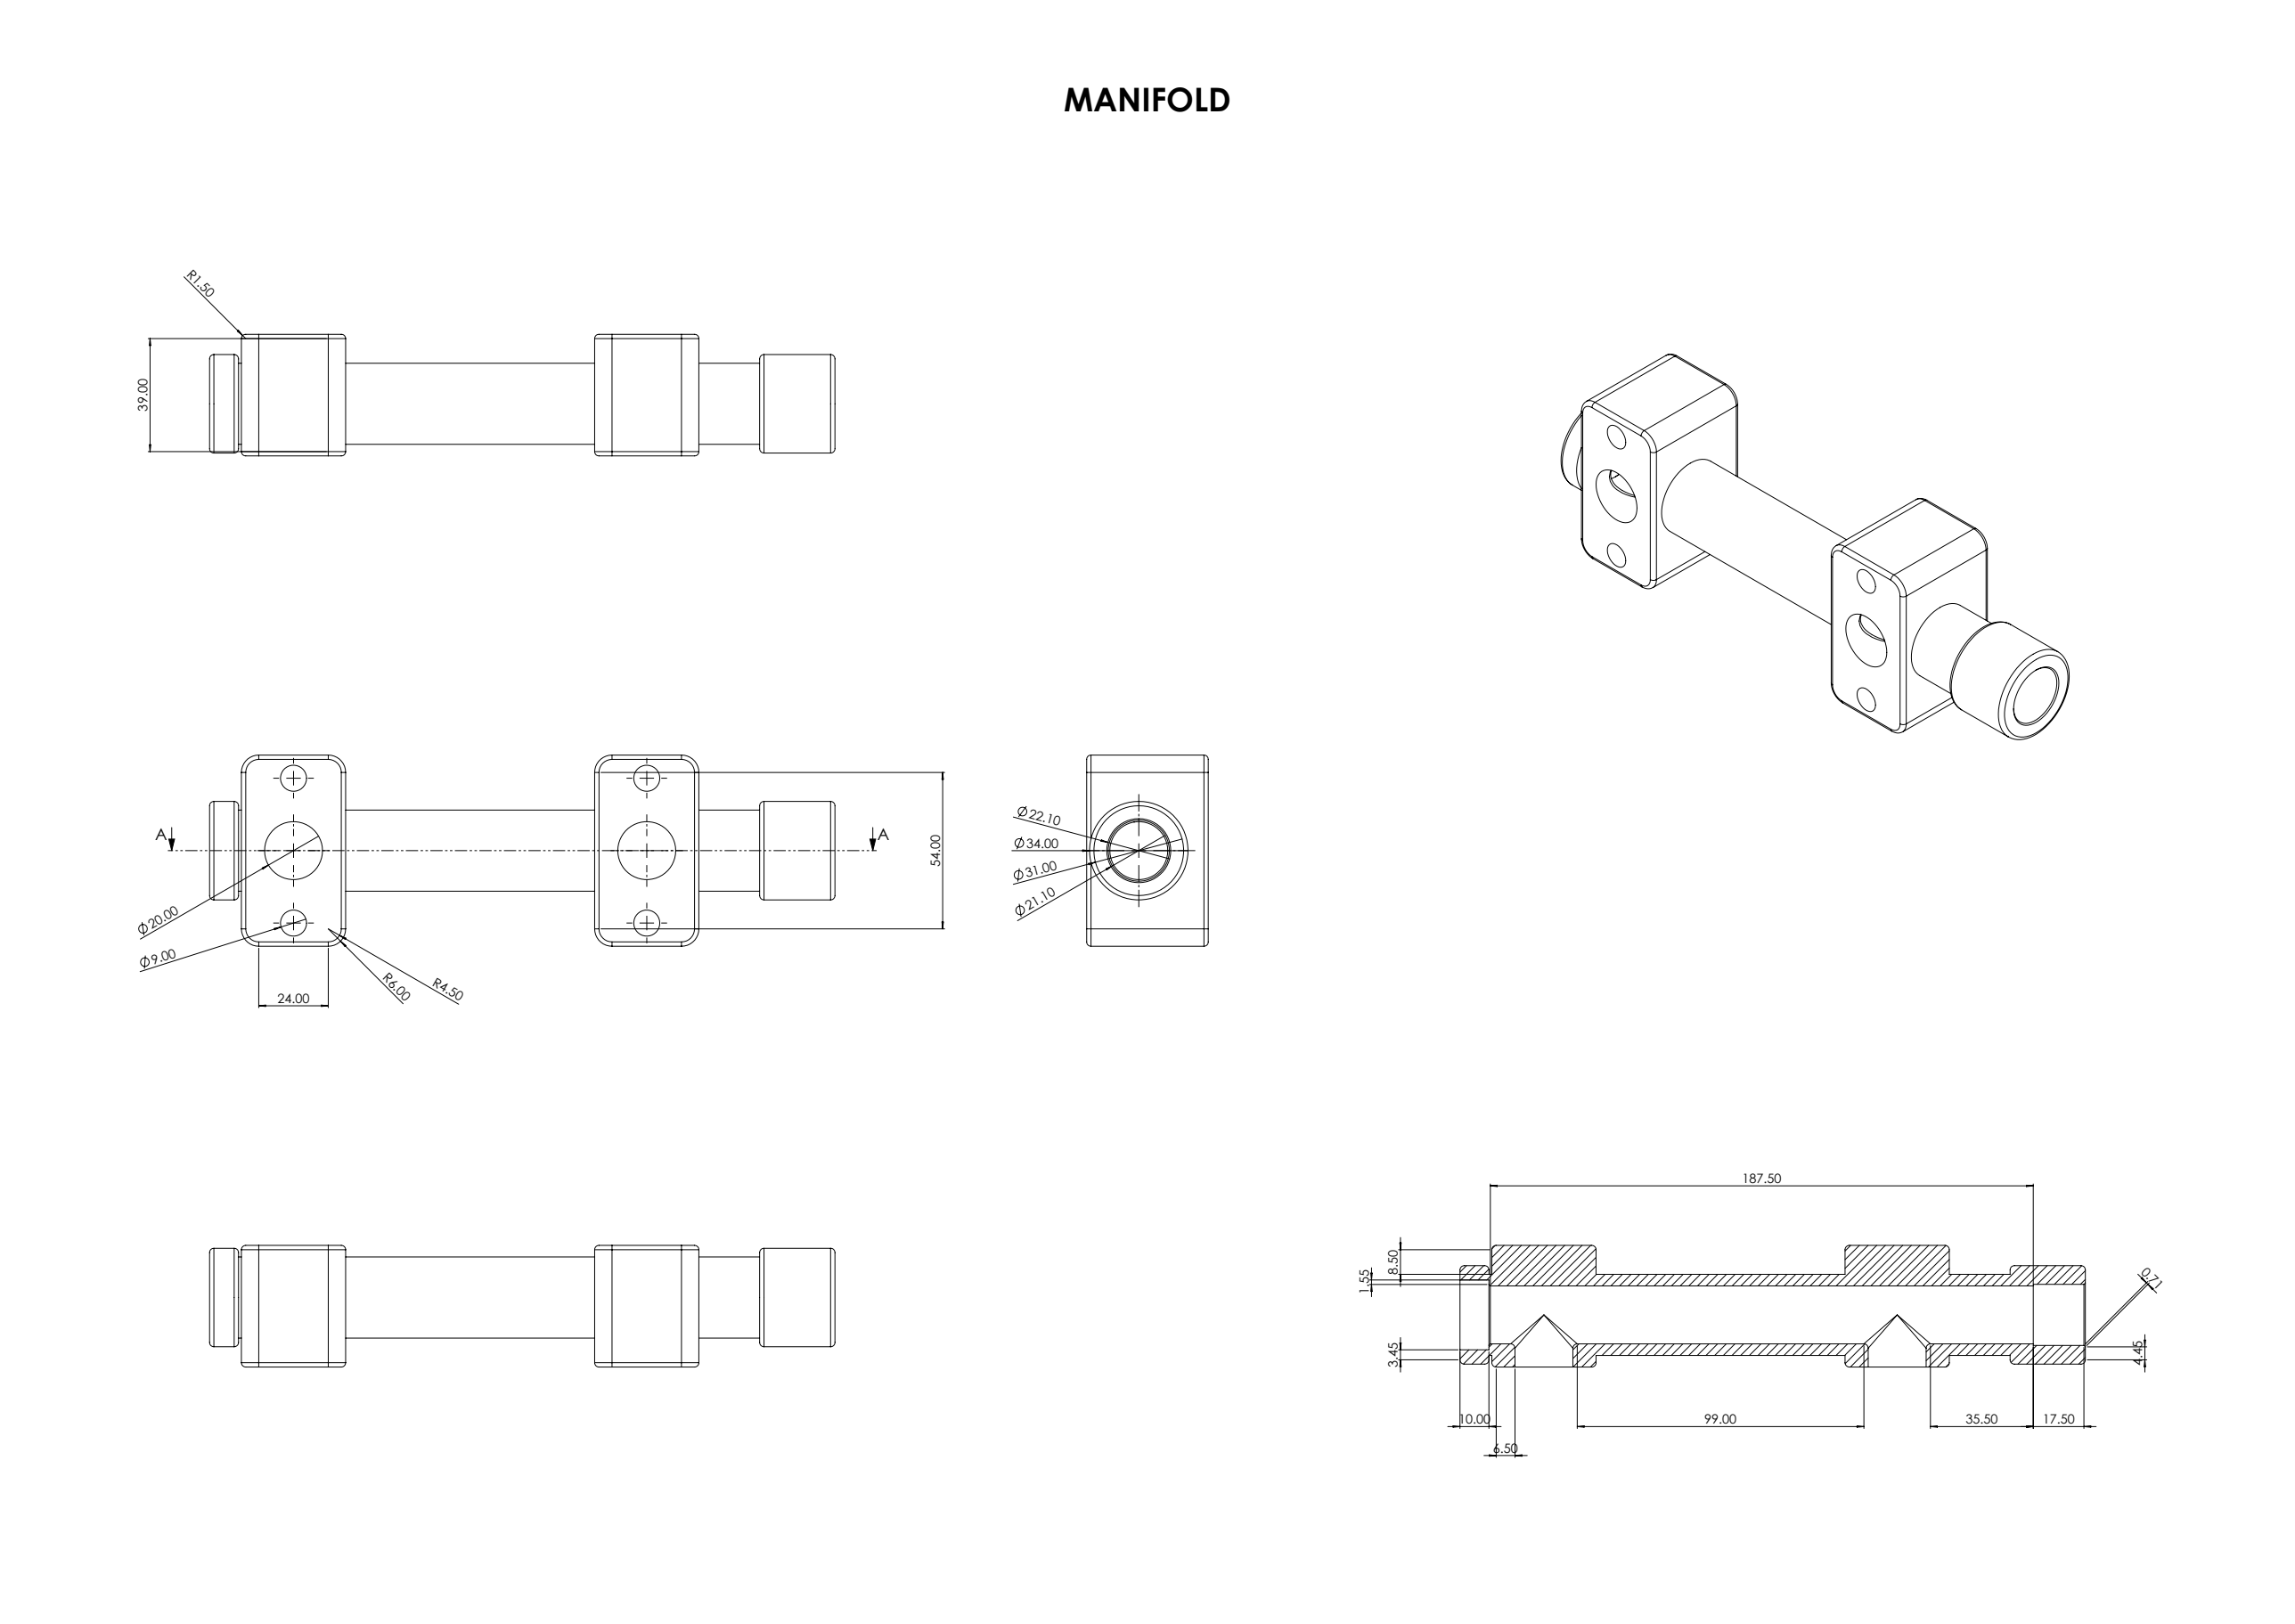
ISO-10303-21;
HEADER;
/* Generated by software containing ST-Developer
 * from STEP Tools, Inc. (www.steptools.com) 
 */

FILE_DESCRIPTION(
/* description */ (''),
/* implementation_level */ '2;1');

FILE_NAME(
/* name */ '10_Manifold.step',
/* time_stamp */ '2026-10-26T06:13:19-07:00',
/* author */ (''),
/* organization */ (''),
/* preprocessor_version */ 'ST-DEVELOPER v20.2',
/* originating_system */ 'Autodesk Translation Framework v15.15.0.0',
/* authorisation */ '');

FILE_SCHEMA (('AUTOMOTIVE_DESIGN { 1 0 10303 214 3 1 1 }','TECHNICAL_DATA_PACKAGING'));
ENDSEC;

DATA;
#10=MECHANICAL_DESIGN_GEOMETRIC_PRESENTATION_REPRESENTATION('',(#306),#56639);
#244=ELLIPSE('',#17827,15.2397506541282,10.);
#245=ELLIPSE('',#17828,15.2397506541282,10.);
#246=ELLIPSE('',#17829,15.2397506541282,10.);
#247=ELLIPSE('',#17830,15.2397506541282,10.);
#248=ELLIPSE('',#17989,15.2397506541282,10.);
#249=ELLIPSE('',#17990,15.2397506541282,10.);
#250=ELLIPSE('',#17991,15.2397506541282,10.);
#251=ELLIPSE('',#17992,15.2397506541282,10.);
#252=ELLIPSE('',#17993,15.2397506541282,10.);
#253=ELLIPSE('',#17994,15.2397506541282,10.);
#266=SHAPE_REPRESENTATION_RELATIONSHIP('SRR','None',#56754,#286);
#286=ADVANCED_BREP_SHAPE_REPRESENTATION('',(#326),#56628);
#306=STYLED_ITEM('',(#56929),#326);
#326=MANIFOLD_SOLID_BREP('Body1',#16958);
#349=B_SPLINE_SURFACE_WITH_KNOTS('',3,3,((#33830,#33831,#33832,#33833,#33834,
#33835,#33836,#33837,#33838,#33839),(#33840,#33841,#33842,#33843,#33844,
#33845,#33846,#33847,#33848,#33849),(#33850,#33851,#33852,#33853,#33854,
#33855,#33856,#33857,#33858,#33859),(#33860,#33861,#33862,#33863,#33864,
#33865,#33866,#33867,#33868,#33869),(#33870,#33871,#33872,#33873,#33874,
#33875,#33876,#33877,#33878,#33879)),.UNSPECIFIED.,.F.,.F.,.F.,(4,1,4),
(4,1,1,1,1,1,1,4),(0.,0.571428571428571,1.),(-1.5707963267949,-1.12199737628207,
-0.673198425769241,-0.224399475256414,0.224399475256414,0.673198425769241,
1.12199737628207,1.5707963267949),.UNSPECIFIED.);
#350=B_SPLINE_SURFACE_WITH_KNOTS('',3,3,((#33883,#33884,#33885,#33886,#33887,
#33888,#33889,#33890,#33891,#33892),(#33893,#33894,#33895,#33896,#33897,
#33898,#33899,#33900,#33901,#33902),(#33903,#33904,#33905,#33906,#33907,
#33908,#33909,#33910,#33911,#33912),(#33913,#33914,#33915,#33916,#33917,
#33918,#33919,#33920,#33921,#33922),(#33923,#33924,#33925,#33926,#33927,
#33928,#33929,#33930,#33931,#33932)),.UNSPECIFIED.,.F.,.F.,.F.,(4,1,4),
(4,1,1,1,1,1,1,4),(0.,0.571428571428571,1.),(-1.5707963267949,-1.12199737628207,
-0.673198425769241,-0.224399475256414,0.224399475256414,0.673198425769241,
1.12199737628207,1.5707963267949),.UNSPECIFIED.);
#351=B_SPLINE_SURFACE_WITH_KNOTS('',3,3,((#33934,#33935,#33936,#33937,#33938,
#33939,#33940,#33941,#33942,#33943),(#33944,#33945,#33946,#33947,#33948,
#33949,#33950,#33951,#33952,#33953),(#33954,#33955,#33956,#33957,#33958,
#33959,#33960,#33961,#33962,#33963),(#33964,#33965,#33966,#33967,#33968,
#33969,#33970,#33971,#33972,#33973),(#33974,#33975,#33976,#33977,#33978,
#33979,#33980,#33981,#33982,#33983)),.UNSPECIFIED.,.F.,.F.,.F.,(4,1,4),
(4,1,1,1,1,1,1,4),(0.,0.571428571428571,1.),(-1.5707963267949,-1.12199737628207,
-0.673198425769241,-0.224399475256414,0.224399475256414,0.673198425769241,
1.12199737628207,1.5707963267949),.UNSPECIFIED.);
#352=B_SPLINE_SURFACE_WITH_KNOTS('',3,3,((#33987,#33988,#33989,#33990,#33991,
#33992,#33993,#33994,#33995,#33996),(#33997,#33998,#33999,#34000,#34001,
#34002,#34003,#34004,#34005,#34006),(#34007,#34008,#34009,#34010,#34011,
#34012,#34013,#34014,#34015,#34016),(#34017,#34018,#34019,#34020,#34021,
#34022,#34023,#34024,#34025,#34026),(#34027,#34028,#34029,#34030,#34031,
#34032,#34033,#34034,#34035,#34036)),.UNSPECIFIED.,.F.,.F.,.F.,(4,1,4),
(4,1,1,1,1,1,1,4),(0.,0.571428571428571,1.),(-1.5707963267949,-1.12199737628207,
-0.673198425769241,-0.224399475256414,0.224399475256414,0.673198425769241,
1.12199737628207,1.5707963267949),.UNSPECIFIED.);
#394=TOROIDAL_SURFACE('',#17838,15.5,1.5);
#395=TOROIDAL_SURFACE('',#17844,15.5,1.5);
#396=TOROIDAL_SURFACE('',#17849,15.5,1.5);
#397=TOROIDAL_SURFACE('',#17858,15.5,1.5);
#398=TOROIDAL_SURFACE('',#17866,4.5,1.5);
#399=TOROIDAL_SURFACE('',#17872,4.50000000000001,1.5);
#400=TOROIDAL_SURFACE('',#17878,4.50000000000001,1.5);
#401=TOROIDAL_SURFACE('',#17884,4.5,1.5);
#402=TOROIDAL_SURFACE('',#17901,4.5,1.5);
#403=TOROIDAL_SURFACE('',#17906,4.50000000000001,1.5);
#404=TOROIDAL_SURFACE('',#17911,4.50000000000001,1.5);
#405=TOROIDAL_SURFACE('',#17917,4.5,1.5);
#406=TOROIDAL_SURFACE('',#17929,4.50000000000001,1.5);
#407=TOROIDAL_SURFACE('',#17935,4.5,1.5);
#408=TOROIDAL_SURFACE('',#17941,4.5,1.5);
#409=TOROIDAL_SURFACE('',#17947,4.50000000000001,1.5);
#410=TOROIDAL_SURFACE('',#17964,4.50000000000001,1.5);
#411=TOROIDAL_SURFACE('',#17969,4.5,1.5);
#412=TOROIDAL_SURFACE('',#17974,4.5,1.5);
#413=TOROIDAL_SURFACE('',#17980,4.50000000000001,1.5);
#514=FACE_BOUND('',#3218,.T.);
#515=FACE_BOUND('',#3222,.T.);
#516=FACE_BOUND('',#3228,.T.);
#517=FACE_BOUND('',#3232,.T.);
#518=FACE_BOUND('',#3235,.T.);
#519=FACE_BOUND('',#3248,.T.);
#520=FACE_BOUND('',#3250,.T.);
#521=FACE_BOUND('',#3251,.T.);
#522=FACE_BOUND('',#3252,.T.);
#523=FACE_BOUND('',#3265,.T.);
#524=FACE_BOUND('',#3266,.T.);
#525=FACE_BOUND('',#3279,.T.);
#526=FACE_BOUND('',#3281,.T.);
#527=FACE_BOUND('',#3282,.T.);
#528=FACE_BOUND('',#3283,.T.);
#529=FACE_BOUND('',#3296,.T.);
#530=FACE_BOUND('',#3297,.T.);
#531=FACE_BOUND('',#3310,.T.);
#532=FACE_BOUND('',#3312,.T.);
#533=FACE_BOUND('',#3315,.T.);
#607=CONICAL_SURFACE('',#17819,10.25,0.785398163397459);
#608=CONICAL_SURFACE('',#17831,10.8,0.785398163397442);
#954=CIRCLE('',#17820,10.5);
#955=CIRCLE('',#17821,10.);
#956=CIRCLE('',#17822,10.);
#957=CIRCLE('',#17824,12.05);
#958=CIRCLE('',#17826,10.);
#959=CIRCLE('',#17832,11.05);
#960=CIRCLE('',#17833,10.55);
#961=CIRCLE('',#17835,15.5);
#962=CIRCLE('',#17837,10.55);
#963=CIRCLE('',#17839,17.);
#964=CIRCLE('',#17840,1.5);
#965=CIRCLE('',#17842,17.);
#966=CIRCLE('',#17843,17.);
#967=CIRCLE('',#17845,1.5);
#968=CIRCLE('',#17846,15.5);
#969=CIRCLE('',#17848,14.);
#970=CIRCLE('',#17850,15.5);
#971=CIRCLE('',#17851,1.5);
#972=CIRCLE('',#17852,17.);
#973=CIRCLE('',#17853,17.);
#974=CIRCLE('',#17855,17.);
#975=CIRCLE('',#17857,14.);
#976=CIRCLE('',#17859,1.5);
#977=CIRCLE('',#17860,15.5);
#978=CIRCLE('',#17862,12.05);
#979=CIRCLE('',#17864,1.5);
#980=CIRCLE('',#17865,1.5);
#981=CIRCLE('',#17867,1.5);
#982=CIRCLE('',#17868,4.5);
#983=CIRCLE('',#17869,6.);
#984=CIRCLE('',#17871,1.5);
#985=CIRCLE('',#17873,1.49999999999999);
#986=CIRCLE('',#17874,4.50000000000001);
#987=CIRCLE('',#17875,6.00000000000001);
#988=CIRCLE('',#17877,1.5);
#989=CIRCLE('',#17879,1.5);
#990=CIRCLE('',#17880,4.50000000000001);
#991=CIRCLE('',#17881,6.00000000000001);
#992=CIRCLE('',#17883,1.5);
#993=CIRCLE('',#17885,4.5);
#994=CIRCLE('',#17886,6.);
#995=CIRCLE('',#17888,6.00000000000001);
#996=CIRCLE('',#17891,6.);
#997=CIRCLE('',#17893,14.);
#998=CIRCLE('',#17895,10.);
#999=CIRCLE('',#17896,4.5);
#1000=CIRCLE('',#17897,4.5);
#1001=CIRCLE('',#17899,1.5);
#1002=CIRCLE('',#17900,1.5);
#1003=CIRCLE('',#17902,1.5);
#1004=CIRCLE('',#17903,4.5);
#1005=CIRCLE('',#17905,1.5);
#1006=CIRCLE('',#17907,1.5);
#1007=CIRCLE('',#17908,4.50000000000001);
#1008=CIRCLE('',#17910,1.5);
#1009=CIRCLE('',#17912,1.5);
#1010=CIRCLE('',#17913,6.00000000000001);
#1011=CIRCLE('',#17914,4.50000000000001);
#1012=CIRCLE('',#17916,1.5);
#1013=CIRCLE('',#17918,6.);
#1014=CIRCLE('',#17919,4.5);
#1015=CIRCLE('',#17924,4.5);
#1016=CIRCLE('',#17925,4.5);
#1017=CIRCLE('',#17927,1.5);
#1018=CIRCLE('',#17928,1.5);
#1019=CIRCLE('',#17930,1.5);
#1020=CIRCLE('',#17931,4.50000000000001);
#1021=CIRCLE('',#17932,6.00000000000001);
#1022=CIRCLE('',#17934,1.5);
#1023=CIRCLE('',#17936,1.49999999999999);
#1024=CIRCLE('',#17937,4.5);
#1025=CIRCLE('',#17938,6.);
#1026=CIRCLE('',#17940,1.5);
#1027=CIRCLE('',#17942,1.5);
#1028=CIRCLE('',#17943,4.5);
#1029=CIRCLE('',#17944,6.);
#1030=CIRCLE('',#17946,1.5);
#1031=CIRCLE('',#17948,4.50000000000001);
#1032=CIRCLE('',#17949,6.00000000000001);
#1033=CIRCLE('',#17951,6.);
#1034=CIRCLE('',#17954,6.00000000000001);
#1035=CIRCLE('',#17956,14.);
#1036=CIRCLE('',#17958,10.);
#1037=CIRCLE('',#17959,4.5);
#1038=CIRCLE('',#17960,4.5);
#1039=CIRCLE('',#17962,1.50000000000001);
#1040=CIRCLE('',#17963,1.5);
#1041=CIRCLE('',#17965,1.5);
#1042=CIRCLE('',#17966,4.50000000000001);
#1043=CIRCLE('',#17968,1.5);
#1044=CIRCLE('',#17970,1.5);
#1045=CIRCLE('',#17971,4.5);
#1046=CIRCLE('',#17973,1.5);
#1047=CIRCLE('',#17975,1.5);
#1048=CIRCLE('',#17976,6.);
#1049=CIRCLE('',#17977,4.5);
#1050=CIRCLE('',#17979,1.5);
#1051=CIRCLE('',#17981,6.00000000000001);
#1052=CIRCLE('',#17982,4.50000000000001);
#1053=CIRCLE('',#17987,4.5);
#1054=CIRCLE('',#17988,4.5);
#1055=CIRCLE('',#18004,14.);
#1056=CIRCLE('',#18007,14.);
#1387=CYLINDRICAL_SURFACE('',#17825,10.);
#1388=CYLINDRICAL_SURFACE('',#17836,10.55);
#1389=CYLINDRICAL_SURFACE('',#17841,17.);
#1390=CYLINDRICAL_SURFACE('',#17854,17.);
#1391=CYLINDRICAL_SURFACE('',#17863,1.5);
#1392=CYLINDRICAL_SURFACE('',#17870,1.5);
#1393=CYLINDRICAL_SURFACE('',#17876,1.5);
#1394=CYLINDRICAL_SURFACE('',#17882,1.5);
#1395=CYLINDRICAL_SURFACE('',#17887,6.00000000000001);
#1396=CYLINDRICAL_SURFACE('',#17890,6.);
#1397=CYLINDRICAL_SURFACE('',#17898,1.5);
#1398=CYLINDRICAL_SURFACE('',#17904,1.5);
#1399=CYLINDRICAL_SURFACE('',#17909,1.5);
#1400=CYLINDRICAL_SURFACE('',#17915,1.5);
#1401=CYLINDRICAL_SURFACE('',#17920,6.00000000000001);
#1402=CYLINDRICAL_SURFACE('',#17922,6.);
#1403=CYLINDRICAL_SURFACE('',#17926,1.5);
#1404=CYLINDRICAL_SURFACE('',#17933,1.5);
#1405=CYLINDRICAL_SURFACE('',#17939,1.5);
#1406=CYLINDRICAL_SURFACE('',#17945,1.5);
#1407=CYLINDRICAL_SURFACE('',#17950,6.);
#1408=CYLINDRICAL_SURFACE('',#17953,6.00000000000001);
#1409=CYLINDRICAL_SURFACE('',#17961,1.5);
#1410=CYLINDRICAL_SURFACE('',#17967,1.5);
#1411=CYLINDRICAL_SURFACE('',#17972,1.5);
#1412=CYLINDRICAL_SURFACE('',#17978,1.5);
#1413=CYLINDRICAL_SURFACE('',#17983,6.);
#1414=CYLINDRICAL_SURFACE('',#17985,6.00000000000001);
#1415=CYLINDRICAL_SURFACE('',#17995,4.5);
#1416=CYLINDRICAL_SURFACE('',#17996,4.5);
#1417=CYLINDRICAL_SURFACE('',#17997,4.5);
#1418=CYLINDRICAL_SURFACE('',#17998,4.5);
#1419=CYLINDRICAL_SURFACE('',#17999,10.);
#1420=CYLINDRICAL_SURFACE('',#18000,10.);
#1421=CYLINDRICAL_SURFACE('',#18001,12.05);
#1422=CYLINDRICAL_SURFACE('',#18005,14.);
#1423=CYLINDRICAL_SURFACE('',#18008,14.);
#1424=CYLINDRICAL_SURFACE('',#18009,14.);
#2143=FACE_OUTER_BOUND('',#3216,.T.);
#2144=FACE_OUTER_BOUND('',#3217,.T.);
#2145=FACE_OUTER_BOUND('',#3219,.T.);
#2146=FACE_OUTER_BOUND('',#3220,.T.);
#2147=FACE_OUTER_BOUND('',#3221,.T.);
#2148=FACE_OUTER_BOUND('',#3223,.T.);
#2149=FACE_OUTER_BOUND('',#3224,.T.);
#2150=FACE_OUTER_BOUND('',#3225,.T.);
#2151=FACE_OUTER_BOUND('',#3226,.T.);
#2152=FACE_OUTER_BOUND('',#3227,.T.);
#2153=FACE_OUTER_BOUND('',#3229,.T.);
#2154=FACE_OUTER_BOUND('',#3230,.T.);
#2155=FACE_OUTER_BOUND('',#3231,.T.);
#2156=FACE_OUTER_BOUND('',#3233,.T.);
#2157=FACE_OUTER_BOUND('',#3234,.T.);
#2158=FACE_OUTER_BOUND('',#3236,.T.);
#2159=FACE_OUTER_BOUND('',#3237,.T.);
#2160=FACE_OUTER_BOUND('',#3238,.T.);
#2161=FACE_OUTER_BOUND('',#3239,.T.);
#2162=FACE_OUTER_BOUND('',#3240,.T.);
#2163=FACE_OUTER_BOUND('',#3241,.T.);
#2164=FACE_OUTER_BOUND('',#3242,.T.);
#2165=FACE_OUTER_BOUND('',#3243,.T.);
#2166=FACE_OUTER_BOUND('',#3244,.T.);
#2167=FACE_OUTER_BOUND('',#3245,.T.);
#2168=FACE_OUTER_BOUND('',#3246,.T.);
#2169=FACE_OUTER_BOUND('',#3247,.T.);
#2170=FACE_OUTER_BOUND('',#3249,.T.);
#2171=FACE_OUTER_BOUND('',#3253,.T.);
#2172=FACE_OUTER_BOUND('',#3254,.T.);
#2173=FACE_OUTER_BOUND('',#3255,.T.);
#2174=FACE_OUTER_BOUND('',#3256,.T.);
#2175=FACE_OUTER_BOUND('',#3257,.T.);
#2176=FACE_OUTER_BOUND('',#3258,.T.);
#2177=FACE_OUTER_BOUND('',#3259,.T.);
#2178=FACE_OUTER_BOUND('',#3260,.T.);
#2179=FACE_OUTER_BOUND('',#3261,.T.);
#2180=FACE_OUTER_BOUND('',#3262,.T.);
#2181=FACE_OUTER_BOUND('',#3263,.T.);
#2182=FACE_OUTER_BOUND('',#3264,.T.);
#2183=FACE_OUTER_BOUND('',#3267,.T.);
#2184=FACE_OUTER_BOUND('',#3268,.T.);
#2185=FACE_OUTER_BOUND('',#3269,.T.);
#2186=FACE_OUTER_BOUND('',#3270,.T.);
#2187=FACE_OUTER_BOUND('',#3271,.T.);
#2188=FACE_OUTER_BOUND('',#3272,.T.);
#2189=FACE_OUTER_BOUND('',#3273,.T.);
#2190=FACE_OUTER_BOUND('',#3274,.T.);
#2191=FACE_OUTER_BOUND('',#3275,.T.);
#2192=FACE_OUTER_BOUND('',#3276,.T.);
#2193=FACE_OUTER_BOUND('',#3277,.T.);
#2194=FACE_OUTER_BOUND('',#3278,.T.);
#2195=FACE_OUTER_BOUND('',#3280,.T.);
#2196=FACE_OUTER_BOUND('',#3284,.T.);
#2197=FACE_OUTER_BOUND('',#3285,.T.);
#2198=FACE_OUTER_BOUND('',#3286,.T.);
#2199=FACE_OUTER_BOUND('',#3287,.T.);
#2200=FACE_OUTER_BOUND('',#3288,.T.);
#2201=FACE_OUTER_BOUND('',#3289,.T.);
#2202=FACE_OUTER_BOUND('',#3290,.T.);
#2203=FACE_OUTER_BOUND('',#3291,.T.);
#2204=FACE_OUTER_BOUND('',#3292,.T.);
#2205=FACE_OUTER_BOUND('',#3293,.T.);
#2206=FACE_OUTER_BOUND('',#3294,.T.);
#2207=FACE_OUTER_BOUND('',#3295,.T.);
#2208=FACE_OUTER_BOUND('',#3298,.T.);
#2209=FACE_OUTER_BOUND('',#3299,.T.);
#2210=FACE_OUTER_BOUND('',#3300,.T.);
#2211=FACE_OUTER_BOUND('',#3301,.T.);
#2212=FACE_OUTER_BOUND('',#3302,.T.);
#2213=FACE_OUTER_BOUND('',#3303,.T.);
#2214=FACE_OUTER_BOUND('',#3304,.T.);
#2215=FACE_OUTER_BOUND('',#3305,.T.);
#2216=FACE_OUTER_BOUND('',#3306,.T.);
#2217=FACE_OUTER_BOUND('',#3307,.T.);
#2218=FACE_OUTER_BOUND('',#3308,.T.);
#2219=FACE_OUTER_BOUND('',#3309,.T.);
#2220=FACE_OUTER_BOUND('',#3311,.T.);
#2221=FACE_OUTER_BOUND('',#3313,.T.);
#2222=FACE_OUTER_BOUND('',#3314,.T.);
#2223=FACE_OUTER_BOUND('',#3316,.T.);
#2224=FACE_OUTER_BOUND('',#3317,.T.);
#3216=EDGE_LOOP('',(#12448,#12449,#12450,#12451,#12452));
#3217=EDGE_LOOP('',(#12453));
#3218=EDGE_LOOP('',(#12454));
#3219=EDGE_LOOP('',(#12455,#12456,#12457,#12458,#12459,#12460,#12461,#12462,
#12463,#12464,#12465,#12466,#12467));
#3220=EDGE_LOOP('',(#12468,#12469,#12470,#12471));
#3221=EDGE_LOOP('',(#12472));
#3222=EDGE_LOOP('',(#12473));
#3223=EDGE_LOOP('',(#12474,#12475,#12476,#12477));
#3224=EDGE_LOOP('',(#12478,#12479,#12480,#12481));
#3225=EDGE_LOOP('',(#12482,#12483,#12484,#12485,#12486));
#3226=EDGE_LOOP('',(#12487,#12488,#12489,#12490,#12491));
#3227=EDGE_LOOP('',(#12492));
#3228=EDGE_LOOP('',(#12493));
#3229=EDGE_LOOP('',(#12494,#12495,#12496,#12497,#12498));
#3230=EDGE_LOOP('',(#12499,#12500,#12501,#12502,#12503));
#3231=EDGE_LOOP('',(#12504));
#3232=EDGE_LOOP('',(#12505));
#3233=EDGE_LOOP('',(#12506,#12507,#12508,#12509));
#3234=EDGE_LOOP('',(#12510));
#3235=EDGE_LOOP('',(#12511));
#3236=EDGE_LOOP('',(#12512,#12513,#12514,#12515));
#3237=EDGE_LOOP('',(#12516,#12517,#12518,#12519));
#3238=EDGE_LOOP('',(#12520,#12521,#12522,#12523));
#3239=EDGE_LOOP('',(#12524,#12525,#12526,#12527));
#3240=EDGE_LOOP('',(#12528,#12529,#12530,#12531));
#3241=EDGE_LOOP('',(#12532,#12533,#12534,#12535));
#3242=EDGE_LOOP('',(#12536,#12537,#12538,#12539));
#3243=EDGE_LOOP('',(#12540,#12541,#12542,#12543));
#3244=EDGE_LOOP('',(#12544,#12545,#12546,#12547));
#3245=EDGE_LOOP('',(#12548,#12549,#12550,#12551));
#3246=EDGE_LOOP('',(#12552,#12553,#12554,#12555));
#3247=EDGE_LOOP('',(#12556,#12557,#12558,#12559));
#3248=EDGE_LOOP('',(#12560));
#3249=EDGE_LOOP('',(#12561,#12562,#12563,#12564,#12565,#12566,#12567,#12568));
#3250=EDGE_LOOP('',(#12569));
#3251=EDGE_LOOP('',(#12570));
#3252=EDGE_LOOP('',(#12571));
#3253=EDGE_LOOP('',(#12572,#12573,#12574,#12575));
#3254=EDGE_LOOP('',(#12576,#12577,#12578,#12579));
#3255=EDGE_LOOP('',(#12580,#12581,#12582,#12583));
#3256=EDGE_LOOP('',(#12584,#12585,#12586,#12587));
#3257=EDGE_LOOP('',(#12588,#12589,#12590,#12591));
#3258=EDGE_LOOP('',(#12592,#12593,#12594,#12595));
#3259=EDGE_LOOP('',(#12596,#12597,#12598,#12599));
#3260=EDGE_LOOP('',(#12600,#12601,#12602,#12603));
#3261=EDGE_LOOP('',(#12604,#12605,#12606,#12607));
#3262=EDGE_LOOP('',(#12608,#12609,#12610,#12611));
#3263=EDGE_LOOP('',(#12612,#12613,#12614,#12615));
#3264=EDGE_LOOP('',(#12616,#12617,#12618,#12619,#12620,#12621,#12622,#12623));
#3265=EDGE_LOOP('',(#12624));
#3266=EDGE_LOOP('',(#12625));
#3267=EDGE_LOOP('',(#12626,#12627,#12628,#12629));
#3268=EDGE_LOOP('',(#12630,#12631,#12632,#12633));
#3269=EDGE_LOOP('',(#12634,#12635,#12636,#12637));
#3270=EDGE_LOOP('',(#12638,#12639,#12640,#12641));
#3271=EDGE_LOOP('',(#12642,#12643,#12644,#12645));
#3272=EDGE_LOOP('',(#12646,#12647,#12648,#12649));
#3273=EDGE_LOOP('',(#12650,#12651,#12652,#12653));
#3274=EDGE_LOOP('',(#12654,#12655,#12656,#12657));
#3275=EDGE_LOOP('',(#12658,#12659,#12660,#12661));
#3276=EDGE_LOOP('',(#12662,#12663,#12664,#12665));
#3277=EDGE_LOOP('',(#12666,#12667,#12668,#12669));
#3278=EDGE_LOOP('',(#12670,#12671,#12672,#12673));
#3279=EDGE_LOOP('',(#12674));
#3280=EDGE_LOOP('',(#12675,#12676,#12677,#12678,#12679,#12680,#12681,#12682));
#3281=EDGE_LOOP('',(#12683));
#3282=EDGE_LOOP('',(#12684));
#3283=EDGE_LOOP('',(#12685));
#3284=EDGE_LOOP('',(#12686,#12687,#12688,#12689));
#3285=EDGE_LOOP('',(#12690,#12691,#12692,#12693));
#3286=EDGE_LOOP('',(#12694,#12695,#12696,#12697));
#3287=EDGE_LOOP('',(#12698,#12699,#12700,#12701));
#3288=EDGE_LOOP('',(#12702,#12703,#12704,#12705));
#3289=EDGE_LOOP('',(#12706,#12707,#12708,#12709));
#3290=EDGE_LOOP('',(#12710,#12711,#12712,#12713));
#3291=EDGE_LOOP('',(#12714,#12715,#12716,#12717));
#3292=EDGE_LOOP('',(#12718,#12719,#12720,#12721));
#3293=EDGE_LOOP('',(#12722,#12723,#12724,#12725));
#3294=EDGE_LOOP('',(#12726,#12727,#12728,#12729));
#3295=EDGE_LOOP('',(#12730,#12731,#12732,#12733,#12734,#12735,#12736,#12737));
#3296=EDGE_LOOP('',(#12738));
#3297=EDGE_LOOP('',(#12739));
#3298=EDGE_LOOP('',(#12740,#12741,#12742));
#3299=EDGE_LOOP('',(#12743,#12744));
#3300=EDGE_LOOP('',(#12745,#12746,#12747));
#3301=EDGE_LOOP('',(#12748,#12749));
#3302=EDGE_LOOP('',(#12750,#12751,#12752,#12753));
#3303=EDGE_LOOP('',(#12754,#12755,#12756,#12757));
#3304=EDGE_LOOP('',(#12758,#12759,#12760,#12761));
#3305=EDGE_LOOP('',(#12762,#12763,#12764,#12765));
#3306=EDGE_LOOP('',(#12766,#12767,#12768,#12769,#12770,#12771));
#3307=EDGE_LOOP('',(#12772,#12773,#12774,#12775,#12776,#12777));
#3308=EDGE_LOOP('',(#12778,#12779,#12780,#12781));
#3309=EDGE_LOOP('',(#12782));
#3310=EDGE_LOOP('',(#12783));
#3311=EDGE_LOOP('',(#12784,#12785,#12786,#12787));
#3312=EDGE_LOOP('',(#12788));
#3313=EDGE_LOOP('',(#12789,#12790,#12791,#12792));
#3314=EDGE_LOOP('',(#12793,#12794,#12795,#12796));
#3315=EDGE_LOOP('',(#12797));
#3316=EDGE_LOOP('',(#12798,#12799,#12800,#12801));
#3317=EDGE_LOOP('',(#12802,#12803,#12804,#12805));
#4189=LINE('',#33507,#5143);
#4190=LINE('',#33516,#5144);
#4191=LINE('',#33518,#5145);
#4192=LINE('',#33520,#5146);
#4193=LINE('',#33532,#5147);
#4194=LINE('',#33540,#5148);
#4195=LINE('',#33547,#5149);
#4196=LINE('',#33568,#5150);
#4197=LINE('',#33585,#5151);
#4198=LINE('',#33588,#5152);
#4199=LINE('',#33599,#5153);
#4200=LINE('',#33600,#5154);
#4201=LINE('',#33611,#5155);
#4202=LINE('',#33612,#5156);
#4203=LINE('',#33623,#5157);
#4204=LINE('',#33624,#5158);
#4205=LINE('',#33630,#5159);
#4206=LINE('',#33633,#5160);
#4207=LINE('',#33636,#5161);
#4208=LINE('',#33637,#5162);
#4209=LINE('',#33640,#5163);
#4210=LINE('',#33644,#5164);
#4211=LINE('',#33645,#5165);
#4212=LINE('',#33659,#5166);
#4213=LINE('',#33668,#5167);
#4214=LINE('',#33677,#5168);
#4215=LINE('',#33678,#5169);
#4216=LINE('',#33689,#5170);
#4217=LINE('',#33690,#5171);
#4218=LINE('',#33695,#5172);
#4219=LINE('',#33696,#5173);
#4220=LINE('',#33698,#5174);
#4221=LINE('',#33710,#5175);
#4222=LINE('',#33713,#5176);
#4223=LINE('',#33724,#5177);
#4224=LINE('',#33725,#5178);
#4225=LINE('',#33736,#5179);
#4226=LINE('',#33737,#5180);
#4227=LINE('',#33748,#5181);
#4228=LINE('',#33749,#5182);
#4229=LINE('',#33755,#5183);
#4230=LINE('',#33758,#5184);
#4231=LINE('',#33761,#5185);
#4232=LINE('',#33762,#5186);
#4233=LINE('',#33765,#5187);
#4234=LINE('',#33769,#5188);
#4235=LINE('',#33770,#5189);
#4236=LINE('',#33784,#5190);
#4237=LINE('',#33793,#5191);
#4238=LINE('',#33802,#5192);
#4239=LINE('',#33803,#5193);
#4240=LINE('',#33814,#5194);
#4241=LINE('',#33815,#5195);
#4242=LINE('',#33820,#5196);
#4243=LINE('',#33821,#5197);
#4244=LINE('',#33823,#5198);
#4245=LINE('',#34039,#5199);
#4246=LINE('',#34041,#5200);
#4247=LINE('',#34043,#5201);
#4248=LINE('',#34045,#5202);
#4249=LINE('',#34047,#5203);
#4250=LINE('',#34049,#5204);
#4251=LINE('',#34051,#5205);
#4252=LINE('',#34057,#5206);
#4253=LINE('',#34062,#5207);
#4254=LINE('',#34064,#5208);
#5143=VECTOR('',#20339,10.25);
#5144=VECTOR('',#20350,10.);
#5145=VECTOR('',#20351,10.);
#5146=VECTOR('',#20352,10.);
#5147=VECTOR('',#20367,10.8);
#5148=VECTOR('',#20378,10.55);
#5149=VECTOR('',#20387,17.);
#5150=VECTOR('',#20414,17.);
#5151=VECTOR('',#20435,10.);
#5152=VECTOR('',#20438,10.);
#5153=VECTOR('',#20451,10.);
#5154=VECTOR('',#20452,10.);
#5155=VECTOR('',#20465,10.);
#5156=VECTOR('',#20466,10.);
#5157=VECTOR('',#20479,10.);
#5158=VECTOR('',#20480,10.);
#5159=VECTOR('',#20489,10.);
#5160=VECTOR('',#20492,10.);
#5161=VECTOR('',#20495,10.);
#5162=VECTOR('',#20496,10.);
#5163=VECTOR('',#20499,10.);
#5164=VECTOR('',#20504,10.);
#5165=VECTOR('',#20505,10.);
#5166=VECTOR('',#20520,10.);
#5167=VECTOR('',#20533,10.);
#5168=VECTOR('',#20544,10.);
#5169=VECTOR('',#20545,10.);
#5170=VECTOR('',#20558,10.);
#5171=VECTOR('',#20559,10.);
#5172=VECTOR('',#20568,10.);
#5173=VECTOR('',#20569,10.);
#5174=VECTOR('',#20572,10.);
#5175=VECTOR('',#20585,10.);
#5176=VECTOR('',#20588,10.);
#5177=VECTOR('',#20601,10.);
#5178=VECTOR('',#20602,10.);
#5179=VECTOR('',#20615,10.);
#5180=VECTOR('',#20616,10.);
#5181=VECTOR('',#20629,10.);
#5182=VECTOR('',#20630,10.);
#5183=VECTOR('',#20639,10.);
#5184=VECTOR('',#20642,10.);
#5185=VECTOR('',#20645,10.);
#5186=VECTOR('',#20646,10.);
#5187=VECTOR('',#20649,10.);
#5188=VECTOR('',#20654,10.);
#5189=VECTOR('',#20655,10.);
#5190=VECTOR('',#20670,10.);
#5191=VECTOR('',#20683,10.);
#5192=VECTOR('',#20694,10.);
#5193=VECTOR('',#20695,10.);
#5194=VECTOR('',#20708,10.);
#5195=VECTOR('',#20709,10.);
#5196=VECTOR('',#20718,10.);
#5197=VECTOR('',#20719,10.);
#5198=VECTOR('',#20722,10.);
#5199=VECTOR('',#20745,4.5);
#5200=VECTOR('',#20748,4.5);
#5201=VECTOR('',#20751,4.5);
#5202=VECTOR('',#20754,4.5);
#5203=VECTOR('',#20757,10.);
#5204=VECTOR('',#20760,10.);
#5205=VECTOR('',#20763,12.05);
#5206=VECTOR('',#20772,14.);
#5207=VECTOR('',#20779,14.);
#5208=VECTOR('',#20782,14.);
#7249=VERTEX_POINT('',#33504);
#7250=VERTEX_POINT('',#33506);
#7251=VERTEX_POINT('',#33508);
#7252=VERTEX_POINT('',#33512);
#7253=VERTEX_POINT('',#33515);
#7254=VERTEX_POINT('',#33517);
#7255=VERTEX_POINT('',#33519);
#7256=VERTEX_POINT('',#33522);
#7257=VERTEX_POINT('',#33525);
#7258=VERTEX_POINT('',#33529);
#7259=VERTEX_POINT('',#33531);
#7260=VERTEX_POINT('',#33535);
#7261=VERTEX_POINT('',#33538);
#7262=VERTEX_POINT('',#33542);
#7263=VERTEX_POINT('',#33546);
#7264=VERTEX_POINT('',#33548);
#7265=VERTEX_POINT('',#33552);
#7266=VERTEX_POINT('',#33556);
#7267=VERTEX_POINT('',#33559);
#7268=VERTEX_POINT('',#33561);
#7269=VERTEX_POINT('',#33563);
#7270=VERTEX_POINT('',#33567);
#7271=VERTEX_POINT('',#33571);
#7272=VERTEX_POINT('',#33574);
#7273=VERTEX_POINT('',#33578);
#7274=VERTEX_POINT('',#33581);
#7275=VERTEX_POINT('',#33582);
#7276=VERTEX_POINT('',#33584);
#7277=VERTEX_POINT('',#33586);
#7278=VERTEX_POINT('',#33590);
#7279=VERTEX_POINT('',#33591);
#7280=VERTEX_POINT('',#33596);
#7281=VERTEX_POINT('',#33597);
#7282=VERTEX_POINT('',#33602);
#7283=VERTEX_POINT('',#33603);
#7284=VERTEX_POINT('',#33608);
#7285=VERTEX_POINT('',#33609);
#7286=VERTEX_POINT('',#33614);
#7287=VERTEX_POINT('',#33615);
#7288=VERTEX_POINT('',#33620);
#7289=VERTEX_POINT('',#33621);
#7290=VERTEX_POINT('',#33629);
#7291=VERTEX_POINT('',#33631);
#7292=VERTEX_POINT('',#33635);
#7293=VERTEX_POINT('',#33639);
#7294=VERTEX_POINT('',#33643);
#7295=VERTEX_POINT('',#33646);
#7296=VERTEX_POINT('',#33649);
#7297=VERTEX_POINT('',#33651);
#7298=VERTEX_POINT('',#33653);
#7299=VERTEX_POINT('',#33656);
#7300=VERTEX_POINT('',#33658);
#7301=VERTEX_POINT('',#33662);
#7302=VERTEX_POINT('',#33666);
#7303=VERTEX_POINT('',#33670);
#7304=VERTEX_POINT('',#33674);
#7305=VERTEX_POINT('',#33675);
#7306=VERTEX_POINT('',#33680);
#7307=VERTEX_POINT('',#33681);
#7308=VERTEX_POINT('',#33686);
#7309=VERTEX_POINT('',#33687);
#7310=VERTEX_POINT('',#33701);
#7311=VERTEX_POINT('',#33703);
#7312=VERTEX_POINT('',#33706);
#7313=VERTEX_POINT('',#33707);
#7314=VERTEX_POINT('',#33709);
#7315=VERTEX_POINT('',#33711);
#7316=VERTEX_POINT('',#33715);
#7317=VERTEX_POINT('',#33716);
#7318=VERTEX_POINT('',#33721);
#7319=VERTEX_POINT('',#33722);
#7320=VERTEX_POINT('',#33727);
#7321=VERTEX_POINT('',#33728);
#7322=VERTEX_POINT('',#33733);
#7323=VERTEX_POINT('',#33734);
#7324=VERTEX_POINT('',#33739);
#7325=VERTEX_POINT('',#33740);
#7326=VERTEX_POINT('',#33745);
#7327=VERTEX_POINT('',#33746);
#7328=VERTEX_POINT('',#33754);
#7329=VERTEX_POINT('',#33756);
#7330=VERTEX_POINT('',#33760);
#7331=VERTEX_POINT('',#33764);
#7332=VERTEX_POINT('',#33768);
#7333=VERTEX_POINT('',#33771);
#7334=VERTEX_POINT('',#33774);
#7335=VERTEX_POINT('',#33776);
#7336=VERTEX_POINT('',#33778);
#7337=VERTEX_POINT('',#33781);
#7338=VERTEX_POINT('',#33783);
#7339=VERTEX_POINT('',#33787);
#7340=VERTEX_POINT('',#33791);
#7341=VERTEX_POINT('',#33795);
#7342=VERTEX_POINT('',#33799);
#7343=VERTEX_POINT('',#33800);
#7344=VERTEX_POINT('',#33805);
#7345=VERTEX_POINT('',#33806);
#7346=VERTEX_POINT('',#33811);
#7347=VERTEX_POINT('',#33812);
#7348=VERTEX_POINT('',#33826);
#7349=VERTEX_POINT('',#33828);
#7350=VERTEX_POINT('',#33880);
#7351=VERTEX_POINT('',#33984);
#7352=VERTEX_POINT('',#34054);
#7353=VERTEX_POINT('',#34059);
#9131=EDGE_CURVE('',#7249,#7249,#954,.T.);
#9132=EDGE_CURVE('',#7249,#7250,#4189,.T.);
#9133=EDGE_CURVE('',#7250,#7251,#955,.T.);
#9134=EDGE_CURVE('',#7251,#7250,#956,.T.);
#9135=EDGE_CURVE('',#7252,#7252,#957,.T.);
#9136=EDGE_CURVE('',#7251,#7253,#4190,.T.);
#9137=EDGE_CURVE('',#7253,#7254,#4191,.T.);
#9138=EDGE_CURVE('',#7254,#7255,#4192,.T.);
#9139=EDGE_CURVE('',#7255,#7255,#958,.T.);
#9140=EDGE_CURVE('',#7256,#7254,#244,.T.);
#9141=EDGE_CURVE('',#7254,#7256,#245,.T.);
#9142=EDGE_CURVE('',#7257,#7253,#246,.T.);
#9143=EDGE_CURVE('',#7253,#7257,#247,.T.);
#9144=EDGE_CURVE('',#7258,#7258,#959,.T.);
#9145=EDGE_CURVE('',#7258,#7259,#4193,.T.);
#9146=EDGE_CURVE('',#7259,#7259,#960,.T.);
#9147=EDGE_CURVE('',#7260,#7260,#961,.T.);
#9148=EDGE_CURVE('',#7261,#7261,#962,.T.);
#9149=EDGE_CURVE('',#7261,#7259,#4194,.T.);
#9150=EDGE_CURVE('',#7262,#7262,#963,.T.);
#9151=EDGE_CURVE('',#7262,#7260,#964,.T.);
#9152=EDGE_CURVE('',#7262,#7263,#4195,.T.);
#9153=EDGE_CURVE('',#7264,#7263,#965,.T.);
#9154=EDGE_CURVE('',#7263,#7264,#966,.T.);
#9155=EDGE_CURVE('',#7264,#7265,#967,.T.);
#9156=EDGE_CURVE('',#7265,#7265,#968,.T.);
#9157=EDGE_CURVE('',#7266,#7266,#969,.T.);
#9158=EDGE_CURVE('',#7267,#7267,#970,.T.);
#9159=EDGE_CURVE('',#7267,#7268,#971,.T.);
#9160=EDGE_CURVE('',#7268,#7269,#972,.T.);
#9161=EDGE_CURVE('',#7269,#7268,#973,.T.);
#9162=EDGE_CURVE('',#7269,#7270,#4196,.T.);
#9163=EDGE_CURVE('',#7270,#7270,#974,.T.);
#9164=EDGE_CURVE('',#7271,#7271,#975,.T.);
#9165=EDGE_CURVE('',#7270,#7272,#976,.T.);
#9166=EDGE_CURVE('',#7272,#7272,#977,.T.);
#9167=EDGE_CURVE('',#7273,#7273,#978,.T.);
#9168=EDGE_CURVE('',#7274,#7275,#979,.T.);
#9169=EDGE_CURVE('',#7275,#7276,#4197,.T.);
#9170=EDGE_CURVE('',#7276,#7277,#980,.T.);
#9171=EDGE_CURVE('',#7277,#7274,#4198,.T.);
#9172=EDGE_CURVE('',#7278,#7279,#981,.T.);
#9173=EDGE_CURVE('',#7279,#7277,#982,.T.);
#9174=EDGE_CURVE('',#7276,#7278,#983,.T.);
#9175=EDGE_CURVE('',#7280,#7281,#984,.T.);
#9176=EDGE_CURVE('',#7281,#7279,#4199,.T.);
#9177=EDGE_CURVE('',#7278,#7280,#4200,.T.);
#9178=EDGE_CURVE('',#7282,#7283,#985,.T.);
#9179=EDGE_CURVE('',#7283,#7281,#986,.T.);
#9180=EDGE_CURVE('',#7280,#7282,#987,.T.);
#9181=EDGE_CURVE('',#7284,#7285,#988,.T.);
#9182=EDGE_CURVE('',#7285,#7283,#4201,.T.);
#9183=EDGE_CURVE('',#7282,#7284,#4202,.T.);
#9184=EDGE_CURVE('',#7286,#7287,#989,.T.);
#9185=EDGE_CURVE('',#7287,#7285,#990,.T.);
#9186=EDGE_CURVE('',#7284,#7286,#991,.T.);
#9187=EDGE_CURVE('',#7288,#7289,#992,.T.);
#9188=EDGE_CURVE('',#7289,#7287,#4203,.T.);
#9189=EDGE_CURVE('',#7286,#7288,#4204,.T.);
#9190=EDGE_CURVE('',#7274,#7289,#993,.T.);
#9191=EDGE_CURVE('',#7288,#7275,#994,.T.);
#9192=EDGE_CURVE('',#7290,#7280,#4205,.T.);
#9193=EDGE_CURVE('',#7291,#7290,#995,.T.);
#9194=EDGE_CURVE('',#7291,#7282,#4206,.T.);
#9195=EDGE_CURVE('',#7292,#7278,#4207,.T.);
#9196=EDGE_CURVE('',#7290,#7292,#4208,.T.);
#9197=EDGE_CURVE('',#7293,#7276,#4209,.T.);
#9198=EDGE_CURVE('',#7292,#7293,#996,.T.);
#9199=EDGE_CURVE('',#7294,#7275,#4210,.T.);
#9200=EDGE_CURVE('',#7293,#7294,#4211,.T.);
#9201=EDGE_CURVE('',#7295,#7295,#997,.T.);
#9202=EDGE_CURVE('',#7296,#7296,#998,.T.);
#9203=EDGE_CURVE('',#7297,#7297,#999,.T.);
#9204=EDGE_CURVE('',#7298,#7298,#1000,.T.);
#9205=EDGE_CURVE('',#7294,#7299,#1001,.T.);
#9206=EDGE_CURVE('',#7299,#7300,#4212,.T.);
#9207=EDGE_CURVE('',#7300,#7293,#1002,.T.);
#9208=EDGE_CURVE('',#7301,#7292,#1003,.T.);
#9209=EDGE_CURVE('',#7300,#7301,#1004,.T.);
#9210=EDGE_CURVE('',#7302,#7290,#1005,.T.);
#9211=EDGE_CURVE('',#7301,#7302,#4213,.T.);
#9212=EDGE_CURVE('',#7303,#7291,#1006,.T.);
#9213=EDGE_CURVE('',#7302,#7303,#1007,.T.);
#9214=EDGE_CURVE('',#7304,#7305,#1008,.T.);
#9215=EDGE_CURVE('',#7305,#7291,#4214,.T.);
#9216=EDGE_CURVE('',#7303,#7304,#4215,.T.);
#9217=EDGE_CURVE('',#7306,#7307,#1009,.T.);
#9218=EDGE_CURVE('',#7307,#7305,#1010,.T.);
#9219=EDGE_CURVE('',#7304,#7306,#1011,.T.);
#9220=EDGE_CURVE('',#7308,#7309,#1012,.T.);
#9221=EDGE_CURVE('',#7309,#7307,#4216,.T.);
#9222=EDGE_CURVE('',#7306,#7308,#4217,.T.);
#9223=EDGE_CURVE('',#7294,#7309,#1013,.T.);
#9224=EDGE_CURVE('',#7308,#7299,#1014,.T.);
#9225=EDGE_CURVE('',#7305,#7284,#4218,.T.);
#9226=EDGE_CURVE('',#7307,#7286,#4219,.T.);
#9227=EDGE_CURVE('',#7309,#7288,#4220,.T.);
#9228=EDGE_CURVE('',#7310,#7310,#1015,.T.);
#9229=EDGE_CURVE('',#7311,#7311,#1016,.T.);
#9230=EDGE_CURVE('',#7312,#7313,#1017,.T.);
#9231=EDGE_CURVE('',#7313,#7314,#4221,.T.);
#9232=EDGE_CURVE('',#7314,#7315,#1018,.T.);
#9233=EDGE_CURVE('',#7315,#7312,#4222,.T.);
#9234=EDGE_CURVE('',#7316,#7317,#1019,.T.);
#9235=EDGE_CURVE('',#7317,#7315,#1020,.T.);
#9236=EDGE_CURVE('',#7314,#7316,#1021,.T.);
#9237=EDGE_CURVE('',#7318,#7319,#1022,.T.);
#9238=EDGE_CURVE('',#7319,#7317,#4223,.T.);
#9239=EDGE_CURVE('',#7316,#7318,#4224,.T.);
#9240=EDGE_CURVE('',#7320,#7321,#1023,.T.);
#9241=EDGE_CURVE('',#7321,#7319,#1024,.T.);
#9242=EDGE_CURVE('',#7318,#7320,#1025,.T.);
#9243=EDGE_CURVE('',#7322,#7323,#1026,.T.);
#9244=EDGE_CURVE('',#7323,#7321,#4225,.T.);
#9245=EDGE_CURVE('',#7320,#7322,#4226,.T.);
#9246=EDGE_CURVE('',#7324,#7325,#1027,.T.);
#9247=EDGE_CURVE('',#7325,#7323,#1028,.T.);
#9248=EDGE_CURVE('',#7322,#7324,#1029,.T.);
#9249=EDGE_CURVE('',#7326,#7327,#1030,.T.);
#9250=EDGE_CURVE('',#7327,#7325,#4227,.T.);
#9251=EDGE_CURVE('',#7324,#7326,#4228,.T.);
#9252=EDGE_CURVE('',#7312,#7327,#1031,.T.);
#9253=EDGE_CURVE('',#7326,#7313,#1032,.T.);
#9254=EDGE_CURVE('',#7328,#7318,#4229,.T.);
#9255=EDGE_CURVE('',#7329,#7328,#1033,.T.);
#9256=EDGE_CURVE('',#7329,#7320,#4230,.T.);
#9257=EDGE_CURVE('',#7330,#7316,#4231,.T.);
#9258=EDGE_CURVE('',#7328,#7330,#4232,.T.);
#9259=EDGE_CURVE('',#7331,#7314,#4233,.T.);
#9260=EDGE_CURVE('',#7330,#7331,#1034,.T.);
#9261=EDGE_CURVE('',#7332,#7313,#4234,.T.);
#9262=EDGE_CURVE('',#7331,#7332,#4235,.T.);
#9263=EDGE_CURVE('',#7333,#7333,#1035,.T.);
#9264=EDGE_CURVE('',#7334,#7334,#1036,.T.);
#9265=EDGE_CURVE('',#7335,#7335,#1037,.T.);
#9266=EDGE_CURVE('',#7336,#7336,#1038,.T.);
#9267=EDGE_CURVE('',#7332,#7337,#1039,.T.);
#9268=EDGE_CURVE('',#7337,#7338,#4236,.T.);
#9269=EDGE_CURVE('',#7338,#7331,#1040,.T.);
#9270=EDGE_CURVE('',#7339,#7330,#1041,.T.);
#9271=EDGE_CURVE('',#7338,#7339,#1042,.T.);
#9272=EDGE_CURVE('',#7340,#7328,#1043,.T.);
#9273=EDGE_CURVE('',#7339,#7340,#4237,.T.);
#9274=EDGE_CURVE('',#7341,#7329,#1044,.T.);
#9275=EDGE_CURVE('',#7340,#7341,#1045,.T.);
#9276=EDGE_CURVE('',#7342,#7343,#1046,.T.);
#9277=EDGE_CURVE('',#7343,#7329,#4238,.T.);
#9278=EDGE_CURVE('',#7341,#7342,#4239,.T.);
#9279=EDGE_CURVE('',#7344,#7345,#1047,.T.);
#9280=EDGE_CURVE('',#7345,#7343,#1048,.T.);
#9281=EDGE_CURVE('',#7342,#7344,#1049,.T.);
#9282=EDGE_CURVE('',#7346,#7347,#1050,.T.);
#9283=EDGE_CURVE('',#7347,#7345,#4240,.T.);
#9284=EDGE_CURVE('',#7344,#7346,#4241,.T.);
#9285=EDGE_CURVE('',#7332,#7347,#1051,.T.);
#9286=EDGE_CURVE('',#7346,#7337,#1052,.T.);
#9287=EDGE_CURVE('',#7343,#7322,#4242,.T.);
#9288=EDGE_CURVE('',#7345,#7324,#4243,.T.);
#9289=EDGE_CURVE('',#7347,#7326,#4244,.T.);
#9290=EDGE_CURVE('',#7348,#7348,#1053,.T.);
#9291=EDGE_CURVE('',#7349,#7349,#1054,.T.);
#9292=EDGE_CURVE('',#7256,#7350,#248,.T.);
#9293=EDGE_CURVE('',#7350,#7254,#249,.T.);
#9294=EDGE_CURVE('',#7254,#7256,#250,.T.);
#9295=EDGE_CURVE('',#7257,#7351,#251,.T.);
#9296=EDGE_CURVE('',#7351,#7253,#252,.T.);
#9297=EDGE_CURVE('',#7253,#7257,#253,.T.);
#9298=EDGE_CURVE('',#7336,#7349,#4245,.T.);
#9299=EDGE_CURVE('',#7298,#7311,#4246,.T.);
#9300=EDGE_CURVE('',#7297,#7310,#4247,.T.);
#9301=EDGE_CURVE('',#7335,#7348,#4248,.T.);
#9302=EDGE_CURVE('',#7296,#7351,#4249,.T.);
#9303=EDGE_CURVE('',#7334,#7350,#4250,.T.);
#9304=EDGE_CURVE('',#7273,#7252,#4251,.T.);
#9305=EDGE_CURVE('',#7352,#7352,#1055,.T.);
#9306=EDGE_CURVE('',#7266,#7352,#4252,.T.);
#9307=EDGE_CURVE('',#7353,#7353,#1056,.T.);
#9308=EDGE_CURVE('',#7333,#7353,#4253,.T.);
#9309=EDGE_CURVE('',#7295,#7271,#4254,.T.);
#12448=ORIENTED_EDGE('',*,*,#9131,.T.);
#12449=ORIENTED_EDGE('',*,*,#9132,.T.);
#12450=ORIENTED_EDGE('',*,*,#9133,.T.);
#12451=ORIENTED_EDGE('',*,*,#9134,.T.);
#12452=ORIENTED_EDGE('',*,*,#9132,.F.);
#12453=ORIENTED_EDGE('',*,*,#9135,.F.);
#12454=ORIENTED_EDGE('',*,*,#9131,.F.);
#12455=ORIENTED_EDGE('',*,*,#9133,.F.);
#12456=ORIENTED_EDGE('',*,*,#9134,.F.);
#12457=ORIENTED_EDGE('',*,*,#9136,.T.);
#12458=ORIENTED_EDGE('',*,*,#9137,.T.);
#12459=ORIENTED_EDGE('',*,*,#9138,.T.);
#12460=ORIENTED_EDGE('',*,*,#9139,.T.);
#12461=ORIENTED_EDGE('',*,*,#9138,.F.);
#12462=ORIENTED_EDGE('',*,*,#9140,.F.);
#12463=ORIENTED_EDGE('',*,*,#9141,.F.);
#12464=ORIENTED_EDGE('',*,*,#9137,.F.);
#12465=ORIENTED_EDGE('',*,*,#9142,.F.);
#12466=ORIENTED_EDGE('',*,*,#9143,.F.);
#12467=ORIENTED_EDGE('',*,*,#9136,.F.);
#12468=ORIENTED_EDGE('',*,*,#9144,.T.);
#12469=ORIENTED_EDGE('',*,*,#9145,.T.);
#12470=ORIENTED_EDGE('',*,*,#9146,.T.);
#12471=ORIENTED_EDGE('',*,*,#9145,.F.);
#12472=ORIENTED_EDGE('',*,*,#9147,.F.);
#12473=ORIENTED_EDGE('',*,*,#9144,.F.);
#12474=ORIENTED_EDGE('',*,*,#9148,.F.);
#12475=ORIENTED_EDGE('',*,*,#9149,.T.);
#12476=ORIENTED_EDGE('',*,*,#9146,.F.);
#12477=ORIENTED_EDGE('',*,*,#9149,.F.);
#12478=ORIENTED_EDGE('',*,*,#9150,.T.);
#12479=ORIENTED_EDGE('',*,*,#9151,.T.);
#12480=ORIENTED_EDGE('',*,*,#9147,.T.);
#12481=ORIENTED_EDGE('',*,*,#9151,.F.);
#12482=ORIENTED_EDGE('',*,*,#9150,.F.);
#12483=ORIENTED_EDGE('',*,*,#9152,.T.);
#12484=ORIENTED_EDGE('',*,*,#9153,.F.);
#12485=ORIENTED_EDGE('',*,*,#9154,.F.);
#12486=ORIENTED_EDGE('',*,*,#9152,.F.);
#12487=ORIENTED_EDGE('',*,*,#9153,.T.);
#12488=ORIENTED_EDGE('',*,*,#9154,.T.);
#12489=ORIENTED_EDGE('',*,*,#9155,.T.);
#12490=ORIENTED_EDGE('',*,*,#9156,.T.);
#12491=ORIENTED_EDGE('',*,*,#9155,.F.);
#12492=ORIENTED_EDGE('',*,*,#9156,.F.);
#12493=ORIENTED_EDGE('',*,*,#9157,.T.);
#12494=ORIENTED_EDGE('',*,*,#9158,.T.);
#12495=ORIENTED_EDGE('',*,*,#9159,.T.);
#12496=ORIENTED_EDGE('',*,*,#9160,.T.);
#12497=ORIENTED_EDGE('',*,*,#9161,.T.);
#12498=ORIENTED_EDGE('',*,*,#9159,.F.);
#12499=ORIENTED_EDGE('',*,*,#9161,.F.);
#12500=ORIENTED_EDGE('',*,*,#9162,.T.);
#12501=ORIENTED_EDGE('',*,*,#9163,.F.);
#12502=ORIENTED_EDGE('',*,*,#9162,.F.);
#12503=ORIENTED_EDGE('',*,*,#9160,.F.);
#12504=ORIENTED_EDGE('',*,*,#9158,.F.);
#12505=ORIENTED_EDGE('',*,*,#9164,.F.);
#12506=ORIENTED_EDGE('',*,*,#9163,.T.);
#12507=ORIENTED_EDGE('',*,*,#9165,.T.);
#12508=ORIENTED_EDGE('',*,*,#9166,.T.);
#12509=ORIENTED_EDGE('',*,*,#9165,.F.);
#12510=ORIENTED_EDGE('',*,*,#9166,.F.);
#12511=ORIENTED_EDGE('',*,*,#9167,.T.);
#12512=ORIENTED_EDGE('',*,*,#9168,.T.);
#12513=ORIENTED_EDGE('',*,*,#9169,.T.);
#12514=ORIENTED_EDGE('',*,*,#9170,.T.);
#12515=ORIENTED_EDGE('',*,*,#9171,.T.);
#12516=ORIENTED_EDGE('',*,*,#9172,.T.);
#12517=ORIENTED_EDGE('',*,*,#9173,.T.);
#12518=ORIENTED_EDGE('',*,*,#9170,.F.);
#12519=ORIENTED_EDGE('',*,*,#9174,.T.);
#12520=ORIENTED_EDGE('',*,*,#9175,.T.);
#12521=ORIENTED_EDGE('',*,*,#9176,.T.);
#12522=ORIENTED_EDGE('',*,*,#9172,.F.);
#12523=ORIENTED_EDGE('',*,*,#9177,.T.);
#12524=ORIENTED_EDGE('',*,*,#9178,.T.);
#12525=ORIENTED_EDGE('',*,*,#9179,.T.);
#12526=ORIENTED_EDGE('',*,*,#9175,.F.);
#12527=ORIENTED_EDGE('',*,*,#9180,.T.);
#12528=ORIENTED_EDGE('',*,*,#9181,.T.);
#12529=ORIENTED_EDGE('',*,*,#9182,.T.);
#12530=ORIENTED_EDGE('',*,*,#9178,.F.);
#12531=ORIENTED_EDGE('',*,*,#9183,.T.);
#12532=ORIENTED_EDGE('',*,*,#9184,.T.);
#12533=ORIENTED_EDGE('',*,*,#9185,.T.);
#12534=ORIENTED_EDGE('',*,*,#9181,.F.);
#12535=ORIENTED_EDGE('',*,*,#9186,.T.);
#12536=ORIENTED_EDGE('',*,*,#9187,.T.);
#12537=ORIENTED_EDGE('',*,*,#9188,.T.);
#12538=ORIENTED_EDGE('',*,*,#9184,.F.);
#12539=ORIENTED_EDGE('',*,*,#9189,.T.);
#12540=ORIENTED_EDGE('',*,*,#9168,.F.);
#12541=ORIENTED_EDGE('',*,*,#9190,.T.);
#12542=ORIENTED_EDGE('',*,*,#9187,.F.);
#12543=ORIENTED_EDGE('',*,*,#9191,.T.);
#12544=ORIENTED_EDGE('',*,*,#9180,.F.);
#12545=ORIENTED_EDGE('',*,*,#9192,.F.);
#12546=ORIENTED_EDGE('',*,*,#9193,.F.);
#12547=ORIENTED_EDGE('',*,*,#9194,.T.);
#12548=ORIENTED_EDGE('',*,*,#9177,.F.);
#12549=ORIENTED_EDGE('',*,*,#9195,.F.);
#12550=ORIENTED_EDGE('',*,*,#9196,.F.);
#12551=ORIENTED_EDGE('',*,*,#9192,.T.);
#12552=ORIENTED_EDGE('',*,*,#9174,.F.);
#12553=ORIENTED_EDGE('',*,*,#9197,.F.);
#12554=ORIENTED_EDGE('',*,*,#9198,.F.);
#12555=ORIENTED_EDGE('',*,*,#9195,.T.);
#12556=ORIENTED_EDGE('',*,*,#9169,.F.);
#12557=ORIENTED_EDGE('',*,*,#9199,.F.);
#12558=ORIENTED_EDGE('',*,*,#9200,.F.);
#12559=ORIENTED_EDGE('',*,*,#9197,.T.);
#12560=ORIENTED_EDGE('',*,*,#9201,.F.);
#12561=ORIENTED_EDGE('',*,*,#9171,.F.);
#12562=ORIENTED_EDGE('',*,*,#9173,.F.);
#12563=ORIENTED_EDGE('',*,*,#9176,.F.);
#12564=ORIENTED_EDGE('',*,*,#9179,.F.);
#12565=ORIENTED_EDGE('',*,*,#9182,.F.);
#12566=ORIENTED_EDGE('',*,*,#9185,.F.);
#12567=ORIENTED_EDGE('',*,*,#9188,.F.);
#12568=ORIENTED_EDGE('',*,*,#9190,.F.);
#12569=ORIENTED_EDGE('',*,*,#9202,.T.);
#12570=ORIENTED_EDGE('',*,*,#9203,.T.);
#12571=ORIENTED_EDGE('',*,*,#9204,.T.);
#12572=ORIENTED_EDGE('',*,*,#9205,.T.);
#12573=ORIENTED_EDGE('',*,*,#9206,.T.);
#12574=ORIENTED_EDGE('',*,*,#9207,.T.);
#12575=ORIENTED_EDGE('',*,*,#9200,.T.);
#12576=ORIENTED_EDGE('',*,*,#9208,.T.);
#12577=ORIENTED_EDGE('',*,*,#9198,.T.);
#12578=ORIENTED_EDGE('',*,*,#9207,.F.);
#12579=ORIENTED_EDGE('',*,*,#9209,.T.);
#12580=ORIENTED_EDGE('',*,*,#9210,.T.);
#12581=ORIENTED_EDGE('',*,*,#9196,.T.);
#12582=ORIENTED_EDGE('',*,*,#9208,.F.);
#12583=ORIENTED_EDGE('',*,*,#9211,.T.);
#12584=ORIENTED_EDGE('',*,*,#9212,.T.);
#12585=ORIENTED_EDGE('',*,*,#9193,.T.);
#12586=ORIENTED_EDGE('',*,*,#9210,.F.);
#12587=ORIENTED_EDGE('',*,*,#9213,.T.);
#12588=ORIENTED_EDGE('',*,*,#9214,.T.);
#12589=ORIENTED_EDGE('',*,*,#9215,.T.);
#12590=ORIENTED_EDGE('',*,*,#9212,.F.);
#12591=ORIENTED_EDGE('',*,*,#9216,.T.);
#12592=ORIENTED_EDGE('',*,*,#9217,.T.);
#12593=ORIENTED_EDGE('',*,*,#9218,.T.);
#12594=ORIENTED_EDGE('',*,*,#9214,.F.);
#12595=ORIENTED_EDGE('',*,*,#9219,.T.);
#12596=ORIENTED_EDGE('',*,*,#9220,.T.);
#12597=ORIENTED_EDGE('',*,*,#9221,.T.);
#12598=ORIENTED_EDGE('',*,*,#9217,.F.);
#12599=ORIENTED_EDGE('',*,*,#9222,.T.);
#12600=ORIENTED_EDGE('',*,*,#9205,.F.);
#12601=ORIENTED_EDGE('',*,*,#9223,.T.);
#12602=ORIENTED_EDGE('',*,*,#9220,.F.);
#12603=ORIENTED_EDGE('',*,*,#9224,.T.);
#12604=ORIENTED_EDGE('',*,*,#9186,.F.);
#12605=ORIENTED_EDGE('',*,*,#9225,.F.);
#12606=ORIENTED_EDGE('',*,*,#9218,.F.);
#12607=ORIENTED_EDGE('',*,*,#9226,.T.);
#12608=ORIENTED_EDGE('',*,*,#9189,.F.);
#12609=ORIENTED_EDGE('',*,*,#9226,.F.);
#12610=ORIENTED_EDGE('',*,*,#9221,.F.);
#12611=ORIENTED_EDGE('',*,*,#9227,.T.);
#12612=ORIENTED_EDGE('',*,*,#9191,.F.);
#12613=ORIENTED_EDGE('',*,*,#9227,.F.);
#12614=ORIENTED_EDGE('',*,*,#9223,.F.);
#12615=ORIENTED_EDGE('',*,*,#9199,.T.);
#12616=ORIENTED_EDGE('',*,*,#9206,.F.);
#12617=ORIENTED_EDGE('',*,*,#9224,.F.);
#12618=ORIENTED_EDGE('',*,*,#9222,.F.);
#12619=ORIENTED_EDGE('',*,*,#9219,.F.);
#12620=ORIENTED_EDGE('',*,*,#9216,.F.);
#12621=ORIENTED_EDGE('',*,*,#9213,.F.);
#12622=ORIENTED_EDGE('',*,*,#9211,.F.);
#12623=ORIENTED_EDGE('',*,*,#9209,.F.);
#12624=ORIENTED_EDGE('',*,*,#9228,.T.);
#12625=ORIENTED_EDGE('',*,*,#9229,.T.);
#12626=ORIENTED_EDGE('',*,*,#9230,.T.);
#12627=ORIENTED_EDGE('',*,*,#9231,.T.);
#12628=ORIENTED_EDGE('',*,*,#9232,.T.);
#12629=ORIENTED_EDGE('',*,*,#9233,.T.);
#12630=ORIENTED_EDGE('',*,*,#9234,.T.);
#12631=ORIENTED_EDGE('',*,*,#9235,.T.);
#12632=ORIENTED_EDGE('',*,*,#9232,.F.);
#12633=ORIENTED_EDGE('',*,*,#9236,.T.);
#12634=ORIENTED_EDGE('',*,*,#9237,.T.);
#12635=ORIENTED_EDGE('',*,*,#9238,.T.);
#12636=ORIENTED_EDGE('',*,*,#9234,.F.);
#12637=ORIENTED_EDGE('',*,*,#9239,.T.);
#12638=ORIENTED_EDGE('',*,*,#9240,.T.);
#12639=ORIENTED_EDGE('',*,*,#9241,.T.);
#12640=ORIENTED_EDGE('',*,*,#9237,.F.);
#12641=ORIENTED_EDGE('',*,*,#9242,.T.);
#12642=ORIENTED_EDGE('',*,*,#9243,.T.);
#12643=ORIENTED_EDGE('',*,*,#9244,.T.);
#12644=ORIENTED_EDGE('',*,*,#9240,.F.);
#12645=ORIENTED_EDGE('',*,*,#9245,.T.);
#12646=ORIENTED_EDGE('',*,*,#9246,.T.);
#12647=ORIENTED_EDGE('',*,*,#9247,.T.);
#12648=ORIENTED_EDGE('',*,*,#9243,.F.);
#12649=ORIENTED_EDGE('',*,*,#9248,.T.);
#12650=ORIENTED_EDGE('',*,*,#9249,.T.);
#12651=ORIENTED_EDGE('',*,*,#9250,.T.);
#12652=ORIENTED_EDGE('',*,*,#9246,.F.);
#12653=ORIENTED_EDGE('',*,*,#9251,.T.);
#12654=ORIENTED_EDGE('',*,*,#9230,.F.);
#12655=ORIENTED_EDGE('',*,*,#9252,.T.);
#12656=ORIENTED_EDGE('',*,*,#9249,.F.);
#12657=ORIENTED_EDGE('',*,*,#9253,.T.);
#12658=ORIENTED_EDGE('',*,*,#9242,.F.);
#12659=ORIENTED_EDGE('',*,*,#9254,.F.);
#12660=ORIENTED_EDGE('',*,*,#9255,.F.);
#12661=ORIENTED_EDGE('',*,*,#9256,.T.);
#12662=ORIENTED_EDGE('',*,*,#9239,.F.);
#12663=ORIENTED_EDGE('',*,*,#9257,.F.);
#12664=ORIENTED_EDGE('',*,*,#9258,.F.);
#12665=ORIENTED_EDGE('',*,*,#9254,.T.);
#12666=ORIENTED_EDGE('',*,*,#9236,.F.);
#12667=ORIENTED_EDGE('',*,*,#9259,.F.);
#12668=ORIENTED_EDGE('',*,*,#9260,.F.);
#12669=ORIENTED_EDGE('',*,*,#9257,.T.);
#12670=ORIENTED_EDGE('',*,*,#9231,.F.);
#12671=ORIENTED_EDGE('',*,*,#9261,.F.);
#12672=ORIENTED_EDGE('',*,*,#9262,.F.);
#12673=ORIENTED_EDGE('',*,*,#9259,.T.);
#12674=ORIENTED_EDGE('',*,*,#9263,.F.);
#12675=ORIENTED_EDGE('',*,*,#9233,.F.);
#12676=ORIENTED_EDGE('',*,*,#9235,.F.);
#12677=ORIENTED_EDGE('',*,*,#9238,.F.);
#12678=ORIENTED_EDGE('',*,*,#9241,.F.);
#12679=ORIENTED_EDGE('',*,*,#9244,.F.);
#12680=ORIENTED_EDGE('',*,*,#9247,.F.);
#12681=ORIENTED_EDGE('',*,*,#9250,.F.);
#12682=ORIENTED_EDGE('',*,*,#9252,.F.);
#12683=ORIENTED_EDGE('',*,*,#9264,.T.);
#12684=ORIENTED_EDGE('',*,*,#9265,.T.);
#12685=ORIENTED_EDGE('',*,*,#9266,.T.);
#12686=ORIENTED_EDGE('',*,*,#9267,.T.);
#12687=ORIENTED_EDGE('',*,*,#9268,.T.);
#12688=ORIENTED_EDGE('',*,*,#9269,.T.);
#12689=ORIENTED_EDGE('',*,*,#9262,.T.);
#12690=ORIENTED_EDGE('',*,*,#9270,.T.);
#12691=ORIENTED_EDGE('',*,*,#9260,.T.);
#12692=ORIENTED_EDGE('',*,*,#9269,.F.);
#12693=ORIENTED_EDGE('',*,*,#9271,.T.);
#12694=ORIENTED_EDGE('',*,*,#9272,.T.);
#12695=ORIENTED_EDGE('',*,*,#9258,.T.);
#12696=ORIENTED_EDGE('',*,*,#9270,.F.);
#12697=ORIENTED_EDGE('',*,*,#9273,.T.);
#12698=ORIENTED_EDGE('',*,*,#9274,.T.);
#12699=ORIENTED_EDGE('',*,*,#9255,.T.);
#12700=ORIENTED_EDGE('',*,*,#9272,.F.);
#12701=ORIENTED_EDGE('',*,*,#9275,.T.);
#12702=ORIENTED_EDGE('',*,*,#9276,.T.);
#12703=ORIENTED_EDGE('',*,*,#9277,.T.);
#12704=ORIENTED_EDGE('',*,*,#9274,.F.);
#12705=ORIENTED_EDGE('',*,*,#9278,.T.);
#12706=ORIENTED_EDGE('',*,*,#9279,.T.);
#12707=ORIENTED_EDGE('',*,*,#9280,.T.);
#12708=ORIENTED_EDGE('',*,*,#9276,.F.);
#12709=ORIENTED_EDGE('',*,*,#9281,.T.);
#12710=ORIENTED_EDGE('',*,*,#9282,.T.);
#12711=ORIENTED_EDGE('',*,*,#9283,.T.);
#12712=ORIENTED_EDGE('',*,*,#9279,.F.);
#12713=ORIENTED_EDGE('',*,*,#9284,.T.);
#12714=ORIENTED_EDGE('',*,*,#9267,.F.);
#12715=ORIENTED_EDGE('',*,*,#9285,.T.);
#12716=ORIENTED_EDGE('',*,*,#9282,.F.);
#12717=ORIENTED_EDGE('',*,*,#9286,.T.);
#12718=ORIENTED_EDGE('',*,*,#9248,.F.);
#12719=ORIENTED_EDGE('',*,*,#9287,.F.);
#12720=ORIENTED_EDGE('',*,*,#9280,.F.);
#12721=ORIENTED_EDGE('',*,*,#9288,.T.);
#12722=ORIENTED_EDGE('',*,*,#9251,.F.);
#12723=ORIENTED_EDGE('',*,*,#9288,.F.);
#12724=ORIENTED_EDGE('',*,*,#9283,.F.);
#12725=ORIENTED_EDGE('',*,*,#9289,.T.);
#12726=ORIENTED_EDGE('',*,*,#9253,.F.);
#12727=ORIENTED_EDGE('',*,*,#9289,.F.);
#12728=ORIENTED_EDGE('',*,*,#9285,.F.);
#12729=ORIENTED_EDGE('',*,*,#9261,.T.);
#12730=ORIENTED_EDGE('',*,*,#9268,.F.);
#12731=ORIENTED_EDGE('',*,*,#9286,.F.);
#12732=ORIENTED_EDGE('',*,*,#9284,.F.);
#12733=ORIENTED_EDGE('',*,*,#9281,.F.);
#12734=ORIENTED_EDGE('',*,*,#9278,.F.);
#12735=ORIENTED_EDGE('',*,*,#9275,.F.);
#12736=ORIENTED_EDGE('',*,*,#9273,.F.);
#12737=ORIENTED_EDGE('',*,*,#9271,.F.);
#12738=ORIENTED_EDGE('',*,*,#9290,.T.);
#12739=ORIENTED_EDGE('',*,*,#9291,.T.);
#12740=ORIENTED_EDGE('',*,*,#9292,.T.);
#12741=ORIENTED_EDGE('',*,*,#9293,.T.);
#12742=ORIENTED_EDGE('',*,*,#9141,.T.);
#12743=ORIENTED_EDGE('',*,*,#9294,.T.);
#12744=ORIENTED_EDGE('',*,*,#9140,.T.);
#12745=ORIENTED_EDGE('',*,*,#9295,.T.);
#12746=ORIENTED_EDGE('',*,*,#9296,.T.);
#12747=ORIENTED_EDGE('',*,*,#9143,.T.);
#12748=ORIENTED_EDGE('',*,*,#9297,.T.);
#12749=ORIENTED_EDGE('',*,*,#9142,.T.);
#12750=ORIENTED_EDGE('',*,*,#9266,.F.);
#12751=ORIENTED_EDGE('',*,*,#9298,.T.);
#12752=ORIENTED_EDGE('',*,*,#9291,.F.);
#12753=ORIENTED_EDGE('',*,*,#9298,.F.);
#12754=ORIENTED_EDGE('',*,*,#9204,.F.);
#12755=ORIENTED_EDGE('',*,*,#9299,.T.);
#12756=ORIENTED_EDGE('',*,*,#9229,.F.);
#12757=ORIENTED_EDGE('',*,*,#9299,.F.);
#12758=ORIENTED_EDGE('',*,*,#9203,.F.);
#12759=ORIENTED_EDGE('',*,*,#9300,.T.);
#12760=ORIENTED_EDGE('',*,*,#9228,.F.);
#12761=ORIENTED_EDGE('',*,*,#9300,.F.);
#12762=ORIENTED_EDGE('',*,*,#9265,.F.);
#12763=ORIENTED_EDGE('',*,*,#9301,.T.);
#12764=ORIENTED_EDGE('',*,*,#9290,.F.);
#12765=ORIENTED_EDGE('',*,*,#9301,.F.);
#12766=ORIENTED_EDGE('',*,*,#9202,.F.);
#12767=ORIENTED_EDGE('',*,*,#9302,.T.);
#12768=ORIENTED_EDGE('',*,*,#9295,.F.);
#12769=ORIENTED_EDGE('',*,*,#9297,.F.);
#12770=ORIENTED_EDGE('',*,*,#9296,.F.);
#12771=ORIENTED_EDGE('',*,*,#9302,.F.);
#12772=ORIENTED_EDGE('',*,*,#9264,.F.);
#12773=ORIENTED_EDGE('',*,*,#9303,.T.);
#12774=ORIENTED_EDGE('',*,*,#9292,.F.);
#12775=ORIENTED_EDGE('',*,*,#9294,.F.);
#12776=ORIENTED_EDGE('',*,*,#9293,.F.);
#12777=ORIENTED_EDGE('',*,*,#9303,.F.);
#12778=ORIENTED_EDGE('',*,*,#9167,.F.);
#12779=ORIENTED_EDGE('',*,*,#9304,.T.);
#12780=ORIENTED_EDGE('',*,*,#9135,.T.);
#12781=ORIENTED_EDGE('',*,*,#9304,.F.);
#12782=ORIENTED_EDGE('',*,*,#9148,.T.);
#12783=ORIENTED_EDGE('',*,*,#9139,.F.);
#12784=ORIENTED_EDGE('',*,*,#9245,.F.);
#12785=ORIENTED_EDGE('',*,*,#9256,.F.);
#12786=ORIENTED_EDGE('',*,*,#9277,.F.);
#12787=ORIENTED_EDGE('',*,*,#9287,.T.);
#12788=ORIENTED_EDGE('',*,*,#9305,.F.);
#12789=ORIENTED_EDGE('',*,*,#9157,.F.);
#12790=ORIENTED_EDGE('',*,*,#9306,.T.);
#12791=ORIENTED_EDGE('',*,*,#9305,.T.);
#12792=ORIENTED_EDGE('',*,*,#9306,.F.);
#12793=ORIENTED_EDGE('',*,*,#9183,.F.);
#12794=ORIENTED_EDGE('',*,*,#9194,.F.);
#12795=ORIENTED_EDGE('',*,*,#9215,.F.);
#12796=ORIENTED_EDGE('',*,*,#9225,.T.);
#12797=ORIENTED_EDGE('',*,*,#9307,.F.);
#12798=ORIENTED_EDGE('',*,*,#9263,.T.);
#12799=ORIENTED_EDGE('',*,*,#9308,.T.);
#12800=ORIENTED_EDGE('',*,*,#9307,.T.);
#12801=ORIENTED_EDGE('',*,*,#9308,.F.);
#12802=ORIENTED_EDGE('',*,*,#9201,.T.);
#12803=ORIENTED_EDGE('',*,*,#9309,.T.);
#12804=ORIENTED_EDGE('',*,*,#9164,.T.);
#12805=ORIENTED_EDGE('',*,*,#9309,.F.);
#15809=PLANE('',#17823);
#15810=PLANE('',#17834);
#15811=PLANE('',#17847);
#15812=PLANE('',#17856);
#15813=PLANE('',#17861);
#15814=PLANE('',#17889);
#15815=PLANE('',#17892);
#15816=PLANE('',#17894);
#15817=PLANE('',#17921);
#15818=PLANE('',#17923);
#15819=PLANE('',#17952);
#15820=PLANE('',#17955);
#15821=PLANE('',#17957);
#15822=PLANE('',#17984);
#15823=PLANE('',#17986);
#15824=PLANE('',#18002);
#15825=PLANE('',#18003);
#15826=PLANE('',#18006);
#16314=ADVANCED_FACE('',(#2143),#607,.F.);
#16315=ADVANCED_FACE('',(#2144,#514),#15809,.F.);
#16316=ADVANCED_FACE('',(#2145),#1387,.F.);
#16317=ADVANCED_FACE('',(#2146),#608,.F.);
#16318=ADVANCED_FACE('',(#2147,#515),#15810,.T.);
#16319=ADVANCED_FACE('',(#2148),#1388,.F.);
#16320=ADVANCED_FACE('',(#2149),#394,.T.);
#16321=ADVANCED_FACE('',(#2150),#1389,.T.);
#16322=ADVANCED_FACE('',(#2151),#395,.T.);
#16323=ADVANCED_FACE('',(#2152,#516),#15811,.T.);
#16324=ADVANCED_FACE('',(#2153),#396,.T.);
#16325=ADVANCED_FACE('',(#2154),#1390,.T.);
#16326=ADVANCED_FACE('',(#2155,#517),#15812,.T.);
#16327=ADVANCED_FACE('',(#2156),#397,.T.);
#16328=ADVANCED_FACE('',(#2157,#518),#15813,.T.);
#16329=ADVANCED_FACE('',(#2158),#1391,.T.);
#16330=ADVANCED_FACE('',(#2159),#398,.T.);
#16331=ADVANCED_FACE('',(#2160),#1392,.T.);
#16332=ADVANCED_FACE('',(#2161),#399,.T.);
#16333=ADVANCED_FACE('',(#2162),#1393,.T.);
#16334=ADVANCED_FACE('',(#2163),#400,.T.);
#16335=ADVANCED_FACE('',(#2164),#1394,.T.);
#16336=ADVANCED_FACE('',(#2165),#401,.T.);
#16337=ADVANCED_FACE('',(#2166),#1395,.T.);
#16338=ADVANCED_FACE('',(#2167),#15814,.T.);
#16339=ADVANCED_FACE('',(#2168),#1396,.T.);
#16340=ADVANCED_FACE('',(#2169,#519),#15815,.T.);
#16341=ADVANCED_FACE('',(#2170,#520,#521,#522),#15816,.T.);
#16342=ADVANCED_FACE('',(#2171),#1397,.T.);
#16343=ADVANCED_FACE('',(#2172),#402,.T.);
#16344=ADVANCED_FACE('',(#2173),#1398,.T.);
#16345=ADVANCED_FACE('',(#2174),#403,.T.);
#16346=ADVANCED_FACE('',(#2175),#1399,.T.);
#16347=ADVANCED_FACE('',(#2176),#404,.T.);
#16348=ADVANCED_FACE('',(#2177),#1400,.T.);
#16349=ADVANCED_FACE('',(#2178),#405,.T.);
#16350=ADVANCED_FACE('',(#2179),#1401,.T.);
#16351=ADVANCED_FACE('',(#2180),#15817,.T.);
#16352=ADVANCED_FACE('',(#2181),#1402,.T.);
#16353=ADVANCED_FACE('',(#2182,#523,#524),#15818,.F.);
#16354=ADVANCED_FACE('',(#2183),#1403,.T.);
#16355=ADVANCED_FACE('',(#2184),#406,.T.);
#16356=ADVANCED_FACE('',(#2185),#1404,.T.);
#16357=ADVANCED_FACE('',(#2186),#407,.T.);
#16358=ADVANCED_FACE('',(#2187),#1405,.T.);
#16359=ADVANCED_FACE('',(#2188),#408,.T.);
#16360=ADVANCED_FACE('',(#2189),#1406,.T.);
#16361=ADVANCED_FACE('',(#2190),#409,.T.);
#16362=ADVANCED_FACE('',(#2191),#1407,.T.);
#16363=ADVANCED_FACE('',(#2192),#15819,.T.);
#16364=ADVANCED_FACE('',(#2193),#1408,.T.);
#16365=ADVANCED_FACE('',(#2194,#525),#15820,.T.);
#16366=ADVANCED_FACE('',(#2195,#526,#527,#528),#15821,.T.);
#16367=ADVANCED_FACE('',(#2196),#1409,.T.);
#16368=ADVANCED_FACE('',(#2197),#410,.T.);
#16369=ADVANCED_FACE('',(#2198),#1410,.T.);
#16370=ADVANCED_FACE('',(#2199),#411,.T.);
#16371=ADVANCED_FACE('',(#2200),#1411,.T.);
#16372=ADVANCED_FACE('',(#2201),#412,.T.);
#16373=ADVANCED_FACE('',(#2202),#1412,.T.);
#16374=ADVANCED_FACE('',(#2203),#413,.T.);
#16375=ADVANCED_FACE('',(#2204),#1413,.T.);
#16376=ADVANCED_FACE('',(#2205),#15822,.T.);
#16377=ADVANCED_FACE('',(#2206),#1414,.T.);
#16378=ADVANCED_FACE('',(#2207,#529,#530),#15823,.F.);
#16379=ADVANCED_FACE('',(#2208),#349,.F.);
#16380=ADVANCED_FACE('',(#2209),#350,.F.);
#16381=ADVANCED_FACE('',(#2210),#351,.F.);
#16382=ADVANCED_FACE('',(#2211),#352,.F.);
#16383=ADVANCED_FACE('',(#2212),#1415,.F.);
#16384=ADVANCED_FACE('',(#2213),#1416,.F.);
#16385=ADVANCED_FACE('',(#2214),#1417,.F.);
#16386=ADVANCED_FACE('',(#2215),#1418,.F.);
#16387=ADVANCED_FACE('',(#2216),#1419,.F.);
#16388=ADVANCED_FACE('',(#2217),#1420,.F.);
#16389=ADVANCED_FACE('',(#2218),#1421,.F.);
#16390=ADVANCED_FACE('',(#2219,#531),#15824,.F.);
#16391=ADVANCED_FACE('',(#2220,#532),#15825,.T.);
#16392=ADVANCED_FACE('',(#2221),#1422,.T.);
#16393=ADVANCED_FACE('',(#2222,#533),#15826,.T.);
#16394=ADVANCED_FACE('',(#2223),#1423,.T.);
#16395=ADVANCED_FACE('',(#2224),#1424,.T.);
#16958=CLOSED_SHELL('',(#16314,#16315,#16316,#16317,#16318,#16319,#16320,
#16321,#16322,#16323,#16324,#16325,#16326,#16327,#16328,#16329,#16330,#16331,
#16332,#16333,#16334,#16335,#16336,#16337,#16338,#16339,#16340,#16341,#16342,
#16343,#16344,#16345,#16346,#16347,#16348,#16349,#16350,#16351,#16352,#16353,
#16354,#16355,#16356,#16357,#16358,#16359,#16360,#16361,#16362,#16363,#16364,
#16365,#16366,#16367,#16368,#16369,#16370,#16371,#16372,#16373,#16374,#16375,
#16376,#16377,#16378,#16379,#16380,#16381,#16382,#16383,#16384,#16385,#16386,
#16387,#16388,#16389,#16390,#16391,#16392,#16393,#16394,#16395));
#17818=AXIS2_PLACEMENT_3D('',#33502,#20333,#20334);
#17819=AXIS2_PLACEMENT_3D('',#33503,#20335,#20336);
#17820=AXIS2_PLACEMENT_3D('',#33505,#20337,#20338);
#17821=AXIS2_PLACEMENT_3D('',#33509,#20340,#20341);
#17822=AXIS2_PLACEMENT_3D('',#33510,#20342,#20343);
#17823=AXIS2_PLACEMENT_3D('',#33511,#20344,#20345);
#17824=AXIS2_PLACEMENT_3D('',#33513,#20346,#20347);
#17825=AXIS2_PLACEMENT_3D('',#33514,#20348,#20349);
#17826=AXIS2_PLACEMENT_3D('',#33521,#20353,#20354);
#17827=AXIS2_PLACEMENT_3D('',#33523,#20355,#20356);
#17828=AXIS2_PLACEMENT_3D('',#33524,#20357,#20358);
#17829=AXIS2_PLACEMENT_3D('',#33526,#20359,#20360);
#17830=AXIS2_PLACEMENT_3D('',#33527,#20361,#20362);
#17831=AXIS2_PLACEMENT_3D('',#33528,#20363,#20364);
#17832=AXIS2_PLACEMENT_3D('',#33530,#20365,#20366);
#17833=AXIS2_PLACEMENT_3D('',#33533,#20368,#20369);
#17834=AXIS2_PLACEMENT_3D('',#33534,#20370,#20371);
#17835=AXIS2_PLACEMENT_3D('',#33536,#20372,#20373);
#17836=AXIS2_PLACEMENT_3D('',#33537,#20374,#20375);
#17837=AXIS2_PLACEMENT_3D('',#33539,#20376,#20377);
#17838=AXIS2_PLACEMENT_3D('',#33541,#20379,#20380);
#17839=AXIS2_PLACEMENT_3D('',#33543,#20381,#20382);
#17840=AXIS2_PLACEMENT_3D('',#33544,#20383,#20384);
#17841=AXIS2_PLACEMENT_3D('',#33545,#20385,#20386);
#17842=AXIS2_PLACEMENT_3D('',#33549,#20388,#20389);
#17843=AXIS2_PLACEMENT_3D('',#33550,#20390,#20391);
#17844=AXIS2_PLACEMENT_3D('',#33551,#20392,#20393);
#17845=AXIS2_PLACEMENT_3D('',#33553,#20394,#20395);
#17846=AXIS2_PLACEMENT_3D('',#33554,#20396,#20397);
#17847=AXIS2_PLACEMENT_3D('',#33555,#20398,#20399);
#17848=AXIS2_PLACEMENT_3D('',#33557,#20400,#20401);
#17849=AXIS2_PLACEMENT_3D('',#33558,#20402,#20403);
#17850=AXIS2_PLACEMENT_3D('',#33560,#20404,#20405);
#17851=AXIS2_PLACEMENT_3D('',#33562,#20406,#20407);
#17852=AXIS2_PLACEMENT_3D('',#33564,#20408,#20409);
#17853=AXIS2_PLACEMENT_3D('',#33565,#20410,#20411);
#17854=AXIS2_PLACEMENT_3D('',#33566,#20412,#20413);
#17855=AXIS2_PLACEMENT_3D('',#33569,#20415,#20416);
#17856=AXIS2_PLACEMENT_3D('',#33570,#20417,#20418);
#17857=AXIS2_PLACEMENT_3D('',#33572,#20419,#20420);
#17858=AXIS2_PLACEMENT_3D('',#33573,#20421,#20422);
#17859=AXIS2_PLACEMENT_3D('',#33575,#20423,#20424);
#17860=AXIS2_PLACEMENT_3D('',#33576,#20425,#20426);
#17861=AXIS2_PLACEMENT_3D('',#33577,#20427,#20428);
#17862=AXIS2_PLACEMENT_3D('',#33579,#20429,#20430);
#17863=AXIS2_PLACEMENT_3D('',#33580,#20431,#20432);
#17864=AXIS2_PLACEMENT_3D('',#33583,#20433,#20434);
#17865=AXIS2_PLACEMENT_3D('',#33587,#20436,#20437);
#17866=AXIS2_PLACEMENT_3D('',#33589,#20439,#20440);
#17867=AXIS2_PLACEMENT_3D('',#33592,#20441,#20442);
#17868=AXIS2_PLACEMENT_3D('',#33593,#20443,#20444);
#17869=AXIS2_PLACEMENT_3D('',#33594,#20445,#20446);
#17870=AXIS2_PLACEMENT_3D('',#33595,#20447,#20448);
#17871=AXIS2_PLACEMENT_3D('',#33598,#20449,#20450);
#17872=AXIS2_PLACEMENT_3D('',#33601,#20453,#20454);
#17873=AXIS2_PLACEMENT_3D('',#33604,#20455,#20456);
#17874=AXIS2_PLACEMENT_3D('',#33605,#20457,#20458);
#17875=AXIS2_PLACEMENT_3D('',#33606,#20459,#20460);
#17876=AXIS2_PLACEMENT_3D('',#33607,#20461,#20462);
#17877=AXIS2_PLACEMENT_3D('',#33610,#20463,#20464);
#17878=AXIS2_PLACEMENT_3D('',#33613,#20467,#20468);
#17879=AXIS2_PLACEMENT_3D('',#33616,#20469,#20470);
#17880=AXIS2_PLACEMENT_3D('',#33617,#20471,#20472);
#17881=AXIS2_PLACEMENT_3D('',#33618,#20473,#20474);
#17882=AXIS2_PLACEMENT_3D('',#33619,#20475,#20476);
#17883=AXIS2_PLACEMENT_3D('',#33622,#20477,#20478);
#17884=AXIS2_PLACEMENT_3D('',#33625,#20481,#20482);
#17885=AXIS2_PLACEMENT_3D('',#33626,#20483,#20484);
#17886=AXIS2_PLACEMENT_3D('',#33627,#20485,#20486);
#17887=AXIS2_PLACEMENT_3D('',#33628,#20487,#20488);
#17888=AXIS2_PLACEMENT_3D('',#33632,#20490,#20491);
#17889=AXIS2_PLACEMENT_3D('',#33634,#20493,#20494);
#17890=AXIS2_PLACEMENT_3D('',#33638,#20497,#20498);
#17891=AXIS2_PLACEMENT_3D('',#33641,#20500,#20501);
#17892=AXIS2_PLACEMENT_3D('',#33642,#20502,#20503);
#17893=AXIS2_PLACEMENT_3D('',#33647,#20506,#20507);
#17894=AXIS2_PLACEMENT_3D('',#33648,#20508,#20509);
#17895=AXIS2_PLACEMENT_3D('',#33650,#20510,#20511);
#17896=AXIS2_PLACEMENT_3D('',#33652,#20512,#20513);
#17897=AXIS2_PLACEMENT_3D('',#33654,#20514,#20515);
#17898=AXIS2_PLACEMENT_3D('',#33655,#20516,#20517);
#17899=AXIS2_PLACEMENT_3D('',#33657,#20518,#20519);
#17900=AXIS2_PLACEMENT_3D('',#33660,#20521,#20522);
#17901=AXIS2_PLACEMENT_3D('',#33661,#20523,#20524);
#17902=AXIS2_PLACEMENT_3D('',#33663,#20525,#20526);
#17903=AXIS2_PLACEMENT_3D('',#33664,#20527,#20528);
#17904=AXIS2_PLACEMENT_3D('',#33665,#20529,#20530);
#17905=AXIS2_PLACEMENT_3D('',#33667,#20531,#20532);
#17906=AXIS2_PLACEMENT_3D('',#33669,#20534,#20535);
#17907=AXIS2_PLACEMENT_3D('',#33671,#20536,#20537);
#17908=AXIS2_PLACEMENT_3D('',#33672,#20538,#20539);
#17909=AXIS2_PLACEMENT_3D('',#33673,#20540,#20541);
#17910=AXIS2_PLACEMENT_3D('',#33676,#20542,#20543);
#17911=AXIS2_PLACEMENT_3D('',#33679,#20546,#20547);
#17912=AXIS2_PLACEMENT_3D('',#33682,#20548,#20549);
#17913=AXIS2_PLACEMENT_3D('',#33683,#20550,#20551);
#17914=AXIS2_PLACEMENT_3D('',#33684,#20552,#20553);
#17915=AXIS2_PLACEMENT_3D('',#33685,#20554,#20555);
#17916=AXIS2_PLACEMENT_3D('',#33688,#20556,#20557);
#17917=AXIS2_PLACEMENT_3D('',#33691,#20560,#20561);
#17918=AXIS2_PLACEMENT_3D('',#33692,#20562,#20563);
#17919=AXIS2_PLACEMENT_3D('',#33693,#20564,#20565);
#17920=AXIS2_PLACEMENT_3D('',#33694,#20566,#20567);
#17921=AXIS2_PLACEMENT_3D('',#33697,#20570,#20571);
#17922=AXIS2_PLACEMENT_3D('',#33699,#20573,#20574);
#17923=AXIS2_PLACEMENT_3D('',#33700,#20575,#20576);
#17924=AXIS2_PLACEMENT_3D('',#33702,#20577,#20578);
#17925=AXIS2_PLACEMENT_3D('',#33704,#20579,#20580);
#17926=AXIS2_PLACEMENT_3D('',#33705,#20581,#20582);
#17927=AXIS2_PLACEMENT_3D('',#33708,#20583,#20584);
#17928=AXIS2_PLACEMENT_3D('',#33712,#20586,#20587);
#17929=AXIS2_PLACEMENT_3D('',#33714,#20589,#20590);
#17930=AXIS2_PLACEMENT_3D('',#33717,#20591,#20592);
#17931=AXIS2_PLACEMENT_3D('',#33718,#20593,#20594);
#17932=AXIS2_PLACEMENT_3D('',#33719,#20595,#20596);
#17933=AXIS2_PLACEMENT_3D('',#33720,#20597,#20598);
#17934=AXIS2_PLACEMENT_3D('',#33723,#20599,#20600);
#17935=AXIS2_PLACEMENT_3D('',#33726,#20603,#20604);
#17936=AXIS2_PLACEMENT_3D('',#33729,#20605,#20606);
#17937=AXIS2_PLACEMENT_3D('',#33730,#20607,#20608);
#17938=AXIS2_PLACEMENT_3D('',#33731,#20609,#20610);
#17939=AXIS2_PLACEMENT_3D('',#33732,#20611,#20612);
#17940=AXIS2_PLACEMENT_3D('',#33735,#20613,#20614);
#17941=AXIS2_PLACEMENT_3D('',#33738,#20617,#20618);
#17942=AXIS2_PLACEMENT_3D('',#33741,#20619,#20620);
#17943=AXIS2_PLACEMENT_3D('',#33742,#20621,#20622);
#17944=AXIS2_PLACEMENT_3D('',#33743,#20623,#20624);
#17945=AXIS2_PLACEMENT_3D('',#33744,#20625,#20626);
#17946=AXIS2_PLACEMENT_3D('',#33747,#20627,#20628);
#17947=AXIS2_PLACEMENT_3D('',#33750,#20631,#20632);
#17948=AXIS2_PLACEMENT_3D('',#33751,#20633,#20634);
#17949=AXIS2_PLACEMENT_3D('',#33752,#20635,#20636);
#17950=AXIS2_PLACEMENT_3D('',#33753,#20637,#20638);
#17951=AXIS2_PLACEMENT_3D('',#33757,#20640,#20641);
#17952=AXIS2_PLACEMENT_3D('',#33759,#20643,#20644);
#17953=AXIS2_PLACEMENT_3D('',#33763,#20647,#20648);
#17954=AXIS2_PLACEMENT_3D('',#33766,#20650,#20651);
#17955=AXIS2_PLACEMENT_3D('',#33767,#20652,#20653);
#17956=AXIS2_PLACEMENT_3D('',#33772,#20656,#20657);
#17957=AXIS2_PLACEMENT_3D('',#33773,#20658,#20659);
#17958=AXIS2_PLACEMENT_3D('',#33775,#20660,#20661);
#17959=AXIS2_PLACEMENT_3D('',#33777,#20662,#20663);
#17960=AXIS2_PLACEMENT_3D('',#33779,#20664,#20665);
#17961=AXIS2_PLACEMENT_3D('',#33780,#20666,#20667);
#17962=AXIS2_PLACEMENT_3D('',#33782,#20668,#20669);
#17963=AXIS2_PLACEMENT_3D('',#33785,#20671,#20672);
#17964=AXIS2_PLACEMENT_3D('',#33786,#20673,#20674);
#17965=AXIS2_PLACEMENT_3D('',#33788,#20675,#20676);
#17966=AXIS2_PLACEMENT_3D('',#33789,#20677,#20678);
#17967=AXIS2_PLACEMENT_3D('',#33790,#20679,#20680);
#17968=AXIS2_PLACEMENT_3D('',#33792,#20681,#20682);
#17969=AXIS2_PLACEMENT_3D('',#33794,#20684,#20685);
#17970=AXIS2_PLACEMENT_3D('',#33796,#20686,#20687);
#17971=AXIS2_PLACEMENT_3D('',#33797,#20688,#20689);
#17972=AXIS2_PLACEMENT_3D('',#33798,#20690,#20691);
#17973=AXIS2_PLACEMENT_3D('',#33801,#20692,#20693);
#17974=AXIS2_PLACEMENT_3D('',#33804,#20696,#20697);
#17975=AXIS2_PLACEMENT_3D('',#33807,#20698,#20699);
#17976=AXIS2_PLACEMENT_3D('',#33808,#20700,#20701);
#17977=AXIS2_PLACEMENT_3D('',#33809,#20702,#20703);
#17978=AXIS2_PLACEMENT_3D('',#33810,#20704,#20705);
#17979=AXIS2_PLACEMENT_3D('',#33813,#20706,#20707);
#17980=AXIS2_PLACEMENT_3D('',#33816,#20710,#20711);
#17981=AXIS2_PLACEMENT_3D('',#33817,#20712,#20713);
#17982=AXIS2_PLACEMENT_3D('',#33818,#20714,#20715);
#17983=AXIS2_PLACEMENT_3D('',#33819,#20716,#20717);
#17984=AXIS2_PLACEMENT_3D('',#33822,#20720,#20721);
#17985=AXIS2_PLACEMENT_3D('',#33824,#20723,#20724);
#17986=AXIS2_PLACEMENT_3D('',#33825,#20725,#20726);
#17987=AXIS2_PLACEMENT_3D('',#33827,#20727,#20728);
#17988=AXIS2_PLACEMENT_3D('',#33829,#20729,#20730);
#17989=AXIS2_PLACEMENT_3D('',#33881,#20731,#20732);
#17990=AXIS2_PLACEMENT_3D('',#33882,#20733,#20734);
#17991=AXIS2_PLACEMENT_3D('',#33933,#20735,#20736);
#17992=AXIS2_PLACEMENT_3D('',#33985,#20737,#20738);
#17993=AXIS2_PLACEMENT_3D('',#33986,#20739,#20740);
#17994=AXIS2_PLACEMENT_3D('',#34037,#20741,#20742);
#17995=AXIS2_PLACEMENT_3D('',#34038,#20743,#20744);
#17996=AXIS2_PLACEMENT_3D('',#34040,#20746,#20747);
#17997=AXIS2_PLACEMENT_3D('',#34042,#20749,#20750);
#17998=AXIS2_PLACEMENT_3D('',#34044,#20752,#20753);
#17999=AXIS2_PLACEMENT_3D('',#34046,#20755,#20756);
#18000=AXIS2_PLACEMENT_3D('',#34048,#20758,#20759);
#18001=AXIS2_PLACEMENT_3D('',#34050,#20761,#20762);
#18002=AXIS2_PLACEMENT_3D('',#34052,#20764,#20765);
#18003=AXIS2_PLACEMENT_3D('',#34053,#20766,#20767);
#18004=AXIS2_PLACEMENT_3D('',#34055,#20768,#20769);
#18005=AXIS2_PLACEMENT_3D('',#34056,#20770,#20771);
#18006=AXIS2_PLACEMENT_3D('',#34058,#20773,#20774);
#18007=AXIS2_PLACEMENT_3D('',#34060,#20775,#20776);
#18008=AXIS2_PLACEMENT_3D('',#34061,#20777,#20778);
#18009=AXIS2_PLACEMENT_3D('',#34063,#20780,#20781);
#20333=DIRECTION('axis',(0.,0.,1.));
#20334=DIRECTION('refdir',(1.,0.,0.));
#20335=DIRECTION('center_axis',(-1.,0.,0.));
#20336=DIRECTION('ref_axis',(0.,-1.,0.));
#20337=DIRECTION('center_axis',(-1.,0.,0.));
#20338=DIRECTION('ref_axis',(0.,-1.,0.));
#20339=DIRECTION('',(0.70710678118654,-0.707106781186555,8.65956056235503E-17));
#20340=DIRECTION('center_axis',(1.,0.,0.));
#20341=DIRECTION('ref_axis',(0.,-1.,0.));
#20342=DIRECTION('center_axis',(1.,0.,0.));
#20343=DIRECTION('ref_axis',(0.,-1.,0.));
#20344=DIRECTION('center_axis',(1.,0.,0.));
#20345=DIRECTION('ref_axis',(0.,0.,-1.));
#20346=DIRECTION('center_axis',(1.,0.,0.));
#20347=DIRECTION('ref_axis',(0.,0.,-1.));
#20348=DIRECTION('center_axis',(1.,0.,0.));
#20349=DIRECTION('ref_axis',(0.,1.,0.));
#20350=DIRECTION('',(1.,0.,0.));
#20351=DIRECTION('',(1.,0.,0.));
#20352=DIRECTION('',(1.,0.,0.));
#20353=DIRECTION('center_axis',(1.,0.,0.));
#20354=DIRECTION('ref_axis',(0.,0.,-1.));
#20355=DIRECTION('center_axis',(0.656178714924787,0.,-0.754605522163505));
#20356=DIRECTION('ref_axis',(0.754605522163505,0.,0.656178714924787));
#20357=DIRECTION('center_axis',(-0.656178714924787,0.,-0.754605522163505));
#20358=DIRECTION('ref_axis',(-0.754605522163505,0.,0.656178714924787));
#20359=DIRECTION('center_axis',(0.656178714924787,0.,-0.754605522163505));
#20360=DIRECTION('ref_axis',(0.754605522163505,0.,0.656178714924787));
#20361=DIRECTION('center_axis',(-0.656178714924787,0.,-0.754605522163505));
#20362=DIRECTION('ref_axis',(-0.754605522163505,0.,0.656178714924787));
#20363=DIRECTION('center_axis',(1.,0.,0.));
#20364=DIRECTION('ref_axis',(0.,1.,0.));
#20365=DIRECTION('center_axis',(1.,0.,0.));
#20366=DIRECTION('ref_axis',(0.,1.,0.));
#20367=DIRECTION('',(-0.707106781186552,0.707106781186543,8.65956056235488E-17));
#20368=DIRECTION('center_axis',(-1.,0.,0.));
#20369=DIRECTION('ref_axis',(0.,1.,0.));
#20370=DIRECTION('center_axis',(1.,0.,0.));
#20371=DIRECTION('ref_axis',(0.,0.,-1.));
#20372=DIRECTION('center_axis',(-1.,0.,0.));
#20373=DIRECTION('ref_axis',(0.,1.,-1.43254583822601E-16));
#20374=DIRECTION('center_axis',(1.,0.,0.));
#20375=DIRECTION('ref_axis',(0.,1.,0.));
#20376=DIRECTION('center_axis',(1.,0.,0.));
#20377=DIRECTION('ref_axis',(0.,0.,-1.));
#20378=DIRECTION('',(1.,0.,0.));
#20379=DIRECTION('center_axis',(-1.,0.,0.));
#20380=DIRECTION('ref_axis',(0.,1.,-1.43254583822601E-16));
#20381=DIRECTION('center_axis',(1.,0.,0.));
#20382=DIRECTION('ref_axis',(0.,1.,-1.43254583822601E-16));
#20383=DIRECTION('center_axis',(0.,2.07899039078655E-17,1.));
#20384=DIRECTION('ref_axis',(0.,-1.,2.07899039078655E-17));
#20385=DIRECTION('center_axis',(1.,0.,0.));
#20386=DIRECTION('ref_axis',(0.,1.,0.));
#20387=DIRECTION('',(-1.,0.,0.));
#20388=DIRECTION('center_axis',(-1.,0.,0.));
#20389=DIRECTION('ref_axis',(0.,-1.,1.83697019872103E-16));
#20390=DIRECTION('center_axis',(-1.,0.,0.));
#20391=DIRECTION('ref_axis',(0.,-1.,1.83697019872103E-16));
#20392=DIRECTION('center_axis',(1.,0.,0.));
#20393=DIRECTION('ref_axis',(0.,0.,-1.));
#20394=DIRECTION('center_axis',(0.,-1.,-1.22464679914735E-16));
#20395=DIRECTION('ref_axis',(0.,-1.22464679914735E-16,1.));
#20396=DIRECTION('center_axis',(1.,0.,0.));
#20397=DIRECTION('ref_axis',(0.,-1.,1.83697019872103E-16));
#20398=DIRECTION('center_axis',(-1.,0.,0.));
#20399=DIRECTION('ref_axis',(0.,0.,1.));
#20400=DIRECTION('center_axis',(1.,0.,0.));
#20401=DIRECTION('ref_axis',(0.,0.,-1.));
#20402=DIRECTION('center_axis',(1.,0.,0.));
#20403=DIRECTION('ref_axis',(0.,0.,-1.));
#20404=DIRECTION('center_axis',(-1.,0.,0.));
#20405=DIRECTION('ref_axis',(0.,-1.,1.83697019872103E-16));
#20406=DIRECTION('center_axis',(0.,-1.,-1.22464679914735E-16));
#20407=DIRECTION('ref_axis',(0.,-1.22464679914735E-16,1.));
#20408=DIRECTION('center_axis',(1.,0.,0.));
#20409=DIRECTION('ref_axis',(0.,-1.,1.83697019872103E-16));
#20410=DIRECTION('center_axis',(1.,0.,0.));
#20411=DIRECTION('ref_axis',(0.,-1.,1.83697019872103E-16));
#20412=DIRECTION('center_axis',(1.,0.,0.));
#20413=DIRECTION('ref_axis',(0.,1.,0.));
#20414=DIRECTION('',(-1.,0.,0.));
#20415=DIRECTION('center_axis',(-1.,0.,0.));
#20416=DIRECTION('ref_axis',(0.,1.,1.22464679914735E-16));
#20417=DIRECTION('center_axis',(1.,0.,0.));
#20418=DIRECTION('ref_axis',(0.,0.,-1.));
#20419=DIRECTION('center_axis',(1.,0.,0.));
#20420=DIRECTION('ref_axis',(0.,0.,-1.));
#20421=DIRECTION('center_axis',(1.,0.,0.));
#20422=DIRECTION('ref_axis',(0.,1.,1.22464679914735E-16));
#20423=DIRECTION('center_axis',(0.,0.,-1.));
#20424=DIRECTION('ref_axis',(0.,-1.,0.));
#20425=DIRECTION('center_axis',(1.,0.,0.));
#20426=DIRECTION('ref_axis',(0.,1.,1.22464679914735E-16));
#20427=DIRECTION('center_axis',(-1.,0.,0.));
#20428=DIRECTION('ref_axis',(0.,0.,1.));
#20429=DIRECTION('center_axis',(1.,0.,0.));
#20430=DIRECTION('ref_axis',(0.,1.,0.));
#20431=DIRECTION('center_axis',(0.,-1.,0.));
#20432=DIRECTION('ref_axis',(-0.707106781186549,0.,0.707106781186546));
#20433=DIRECTION('center_axis',(0.,-1.,0.));
#20434=DIRECTION('ref_axis',(0.,0.,1.));
#20435=DIRECTION('',(0.,-1.,0.));
#20436=DIRECTION('center_axis',(2.96059473233374E-15,1.,0.));
#20437=DIRECTION('ref_axis',(-1.,2.96059473233374E-15,1.48029736616687E-15));
#20438=DIRECTION('',(0.,1.,0.));
#20439=DIRECTION('center_axis',(0.,0.,1.));
#20440=DIRECTION('ref_axis',(1.,0.,0.));
#20441=DIRECTION('center_axis',(-1.,0.,0.));
#20442=DIRECTION('ref_axis',(0.,-1.,0.));
#20443=DIRECTION('center_axis',(0.,0.,-1.));
#20444=DIRECTION('ref_axis',(-0.707106781186547,-0.707106781186548,0.));
#20445=DIRECTION('center_axis',(0.,0.,1.));
#20446=DIRECTION('ref_axis',(-0.707106781186547,-0.707106781186548,0.));
#20447=DIRECTION('center_axis',(1.,0.,0.));
#20448=DIRECTION('ref_axis',(0.,-0.707106781186547,0.707106781186548));
#20449=DIRECTION('center_axis',(-1.,0.,0.));
#20450=DIRECTION('ref_axis',(0.,-1.,1.48029736616688E-15));
#20451=DIRECTION('',(-1.,0.,0.));
#20452=DIRECTION('',(1.,0.,0.));
#20453=DIRECTION('center_axis',(0.,0.,1.));
#20454=DIRECTION('ref_axis',(1.,0.,0.));
#20455=DIRECTION('center_axis',(-2.96059473233376E-15,-1.,0.));
#20456=DIRECTION('ref_axis',(1.,-2.96059473233376E-15,0.));
#20457=DIRECTION('center_axis',(0.,0.,-1.));
#20458=DIRECTION('ref_axis',(0.707106781186547,-0.707106781186548,0.));
#20459=DIRECTION('center_axis',(0.,0.,1.));
#20460=DIRECTION('ref_axis',(0.707106781186547,-0.707106781186548,0.));
#20461=DIRECTION('center_axis',(0.,1.,0.));
#20462=DIRECTION('ref_axis',(0.707106781186549,0.,0.707106781186546));
#20463=DIRECTION('center_axis',(-2.96059473233374E-15,-1.,0.));
#20464=DIRECTION('ref_axis',(1.,-2.96059473233374E-15,1.48029736616687E-15));
#20465=DIRECTION('',(0.,-1.,0.));
#20466=DIRECTION('',(0.,1.,0.));
#20467=DIRECTION('center_axis',(0.,0.,1.));
#20468=DIRECTION('ref_axis',(1.,0.,0.));
#20469=DIRECTION('center_axis',(1.,0.,0.));
#20470=DIRECTION('ref_axis',(0.,1.,0.));
#20471=DIRECTION('center_axis',(0.,0.,-1.));
#20472=DIRECTION('ref_axis',(0.707106781186547,0.707106781186548,0.));
#20473=DIRECTION('center_axis',(0.,0.,1.));
#20474=DIRECTION('ref_axis',(0.707106781186547,0.707106781186548,0.));
#20475=DIRECTION('center_axis',(-1.,0.,0.));
#20476=DIRECTION('ref_axis',(0.,0.707106781186547,0.707106781186548));
#20477=DIRECTION('center_axis',(1.,0.,0.));
#20478=DIRECTION('ref_axis',(0.,1.,1.48029736616688E-15));
#20479=DIRECTION('',(1.,0.,0.));
#20480=DIRECTION('',(-1.,0.,0.));
#20481=DIRECTION('center_axis',(0.,0.,1.));
#20482=DIRECTION('ref_axis',(1.,0.,0.));
#20483=DIRECTION('center_axis',(0.,0.,-1.));
#20484=DIRECTION('ref_axis',(-0.707106781186547,0.707106781186548,0.));
#20485=DIRECTION('center_axis',(0.,0.,1.));
#20486=DIRECTION('ref_axis',(-0.707106781186547,0.707106781186548,0.));
#20487=DIRECTION('center_axis',(0.,0.,1.));
#20488=DIRECTION('ref_axis',(1.48029736616687E-15,-1.,0.));
#20489=DIRECTION('',(0.,0.,1.));
#20490=DIRECTION('center_axis',(0.,0.,-1.));
#20491=DIRECTION('ref_axis',(0.707106781186547,-0.707106781186548,0.));
#20492=DIRECTION('',(0.,0.,1.));
#20493=DIRECTION('center_axis',(0.,-1.,0.));
#20494=DIRECTION('ref_axis',(1.,0.,0.));
#20495=DIRECTION('',(0.,0.,1.));
#20496=DIRECTION('',(-1.,0.,0.));
#20497=DIRECTION('center_axis',(0.,0.,1.));
#20498=DIRECTION('ref_axis',(-1.,0.,0.));
#20499=DIRECTION('',(0.,0.,1.));
#20500=DIRECTION('center_axis',(0.,0.,-1.));
#20501=DIRECTION('ref_axis',(-0.707106781186547,-0.707106781186548,0.));
#20502=DIRECTION('center_axis',(-1.,0.,0.));
#20503=DIRECTION('ref_axis',(0.,-1.,0.));
#20504=DIRECTION('',(0.,0.,1.));
#20505=DIRECTION('',(0.,1.,0.));
#20506=DIRECTION('center_axis',(-1.,0.,0.));
#20507=DIRECTION('ref_axis',(0.,1.,0.));
#20508=DIRECTION('center_axis',(0.,0.,1.));
#20509=DIRECTION('ref_axis',(1.,0.,0.));
#20510=DIRECTION('center_axis',(0.,0.,-1.));
#20511=DIRECTION('ref_axis',(1.,0.,0.));
#20512=DIRECTION('center_axis',(0.,0.,-1.));
#20513=DIRECTION('ref_axis',(1.,0.,0.));
#20514=DIRECTION('center_axis',(0.,0.,-1.));
#20515=DIRECTION('ref_axis',(1.,0.,0.));
#20516=DIRECTION('center_axis',(0.,-1.,0.));
#20517=DIRECTION('ref_axis',(-0.707106781186548,0.,-0.707106781186548));
#20518=DIRECTION('center_axis',(0.,-1.,0.));
#20519=DIRECTION('ref_axis',(-1.,0.,0.));
#20520=DIRECTION('',(0.,-1.,0.));
#20521=DIRECTION('center_axis',(2.96059473233374E-15,1.,0.));
#20522=DIRECTION('ref_axis',(0.,0.,-1.));
#20523=DIRECTION('center_axis',(0.,0.,1.));
#20524=DIRECTION('ref_axis',(1.,0.,0.));
#20525=DIRECTION('center_axis',(-1.,0.,0.));
#20526=DIRECTION('ref_axis',(0.,0.,-1.));
#20527=DIRECTION('center_axis',(0.,0.,1.));
#20528=DIRECTION('ref_axis',(-0.707106781186547,-0.707106781186548,0.));
#20529=DIRECTION('center_axis',(1.,0.,0.));
#20530=DIRECTION('ref_axis',(0.,-0.707106781186545,-0.70710678118655));
#20531=DIRECTION('center_axis',(-1.,0.,0.));
#20532=DIRECTION('ref_axis',(0.,0.,-1.));
#20533=DIRECTION('',(1.,0.,0.));
#20534=DIRECTION('center_axis',(0.,0.,1.));
#20535=DIRECTION('ref_axis',(1.,0.,0.));
#20536=DIRECTION('center_axis',(-2.96059473233376E-15,-1.,0.));
#20537=DIRECTION('ref_axis',(0.,0.,-1.));
#20538=DIRECTION('center_axis',(0.,0.,1.));
#20539=DIRECTION('ref_axis',(0.707106781186547,-0.707106781186548,0.));
#20540=DIRECTION('center_axis',(0.,1.,0.));
#20541=DIRECTION('ref_axis',(0.707106781186552,0.,-0.707106781186543));
#20542=DIRECTION('center_axis',(-2.96059473233373E-15,-1.,0.));
#20543=DIRECTION('ref_axis',(0.,0.,-1.));
#20544=DIRECTION('',(0.,-1.,0.));
#20545=DIRECTION('',(0.,1.,0.));
#20546=DIRECTION('center_axis',(0.,0.,1.));
#20547=DIRECTION('ref_axis',(1.,0.,0.));
#20548=DIRECTION('center_axis',(1.,0.,0.));
#20549=DIRECTION('ref_axis',(0.,0.,-1.));
#20550=DIRECTION('center_axis',(0.,0.,-1.));
#20551=DIRECTION('ref_axis',(0.707106781186547,0.707106781186548,0.));
#20552=DIRECTION('center_axis',(0.,0.,1.));
#20553=DIRECTION('ref_axis',(0.707106781186547,0.707106781186548,0.));
#20554=DIRECTION('center_axis',(-1.,0.,0.));
#20555=DIRECTION('ref_axis',(0.,0.707106781186545,-0.70710678118655));
#20556=DIRECTION('center_axis',(1.,0.,0.));
#20557=DIRECTION('ref_axis',(0.,0.,-1.));
#20558=DIRECTION('',(1.,0.,0.));
#20559=DIRECTION('',(-1.,0.,0.));
#20560=DIRECTION('center_axis',(0.,0.,1.));
#20561=DIRECTION('ref_axis',(1.,0.,0.));
#20562=DIRECTION('center_axis',(0.,0.,-1.));
#20563=DIRECTION('ref_axis',(-0.707106781186547,0.707106781186548,0.));
#20564=DIRECTION('center_axis',(0.,0.,1.));
#20565=DIRECTION('ref_axis',(-0.707106781186547,0.707106781186548,0.));
#20566=DIRECTION('center_axis',(0.,0.,1.));
#20567=DIRECTION('ref_axis',(1.,2.96059473233374E-15,0.));
#20568=DIRECTION('',(0.,0.,1.));
#20569=DIRECTION('',(0.,0.,1.));
#20570=DIRECTION('center_axis',(0.,1.,0.));
#20571=DIRECTION('ref_axis',(-1.,0.,0.));
#20572=DIRECTION('',(0.,0.,1.));
#20573=DIRECTION('center_axis',(0.,0.,1.));
#20574=DIRECTION('ref_axis',(1.48029736616688E-15,1.,0.));
#20575=DIRECTION('center_axis',(0.,0.,1.));
#20576=DIRECTION('ref_axis',(1.,0.,0.));
#20577=DIRECTION('center_axis',(0.,0.,1.));
#20578=DIRECTION('ref_axis',(1.,0.,0.));
#20579=DIRECTION('center_axis',(0.,0.,1.));
#20580=DIRECTION('ref_axis',(1.,0.,0.));
#20581=DIRECTION('center_axis',(0.,-1.,0.));
#20582=DIRECTION('ref_axis',(-0.707106781186549,0.,0.707106781186546));
#20583=DIRECTION('center_axis',(0.,-1.,0.));
#20584=DIRECTION('ref_axis',(0.,0.,1.));
#20585=DIRECTION('',(0.,-1.,0.));
#20586=DIRECTION('center_axis',(2.96059473233374E-15,1.,0.));
#20587=DIRECTION('ref_axis',(-1.,2.96059473233374E-15,1.48029736616687E-15));
#20588=DIRECTION('',(0.,1.,0.));
#20589=DIRECTION('center_axis',(0.,0.,1.));
#20590=DIRECTION('ref_axis',(1.,0.,0.));
#20591=DIRECTION('center_axis',(-1.,0.,0.));
#20592=DIRECTION('ref_axis',(0.,-1.,0.));
#20593=DIRECTION('center_axis',(0.,0.,-1.));
#20594=DIRECTION('ref_axis',(-0.707106781186547,-0.707106781186548,0.));
#20595=DIRECTION('center_axis',(0.,0.,1.));
#20596=DIRECTION('ref_axis',(-0.707106781186547,-0.707106781186548,0.));
#20597=DIRECTION('center_axis',(1.,0.,0.));
#20598=DIRECTION('ref_axis',(0.,-0.707106781186547,0.707106781186548));
#20599=DIRECTION('center_axis',(-1.,0.,0.));
#20600=DIRECTION('ref_axis',(0.,-1.,1.48029736616688E-15));
#20601=DIRECTION('',(-1.,0.,0.));
#20602=DIRECTION('',(1.,0.,0.));
#20603=DIRECTION('center_axis',(0.,0.,1.));
#20604=DIRECTION('ref_axis',(1.,0.,0.));
#20605=DIRECTION('center_axis',(0.,-1.,0.));
#20606=DIRECTION('ref_axis',(1.,0.,0.));
#20607=DIRECTION('center_axis',(0.,0.,-1.));
#20608=DIRECTION('ref_axis',(0.707106781186547,-0.707106781186548,0.));
#20609=DIRECTION('center_axis',(0.,0.,1.));
#20610=DIRECTION('ref_axis',(0.707106781186547,-0.707106781186548,0.));
#20611=DIRECTION('center_axis',(0.,1.,0.));
#20612=DIRECTION('ref_axis',(0.707106781186549,0.,0.707106781186546));
#20613=DIRECTION('center_axis',(-2.96059473233374E-15,-1.,0.));
#20614=DIRECTION('ref_axis',(1.,-2.96059473233374E-15,1.48029736616687E-15));
#20615=DIRECTION('',(0.,-1.,0.));
#20616=DIRECTION('',(0.,1.,0.));
#20617=DIRECTION('center_axis',(0.,0.,1.));
#20618=DIRECTION('ref_axis',(1.,0.,0.));
#20619=DIRECTION('center_axis',(1.,0.,0.));
#20620=DIRECTION('ref_axis',(0.,1.,0.));
#20621=DIRECTION('center_axis',(0.,0.,-1.));
#20622=DIRECTION('ref_axis',(0.707106781186547,0.707106781186548,0.));
#20623=DIRECTION('center_axis',(0.,0.,1.));
#20624=DIRECTION('ref_axis',(0.707106781186547,0.707106781186548,0.));
#20625=DIRECTION('center_axis',(-1.,0.,0.));
#20626=DIRECTION('ref_axis',(0.,0.707106781186547,0.707106781186548));
#20627=DIRECTION('center_axis',(1.,0.,0.));
#20628=DIRECTION('ref_axis',(0.,1.,1.48029736616688E-15));
#20629=DIRECTION('',(1.,0.,0.));
#20630=DIRECTION('',(-1.,0.,0.));
#20631=DIRECTION('center_axis',(0.,0.,1.));
#20632=DIRECTION('ref_axis',(1.,0.,0.));
#20633=DIRECTION('center_axis',(0.,0.,-1.));
#20634=DIRECTION('ref_axis',(-0.707106781186547,0.707106781186548,0.));
#20635=DIRECTION('center_axis',(0.,0.,1.));
#20636=DIRECTION('ref_axis',(-0.707106781186547,0.707106781186548,0.));
#20637=DIRECTION('center_axis',(0.,0.,1.));
#20638=DIRECTION('ref_axis',(-1.48029736616688E-15,-1.,0.));
#20639=DIRECTION('',(0.,0.,1.));
#20640=DIRECTION('center_axis',(0.,0.,-1.));
#20641=DIRECTION('ref_axis',(0.707106781186547,-0.707106781186548,0.));
#20642=DIRECTION('',(0.,0.,1.));
#20643=DIRECTION('center_axis',(0.,-1.,0.));
#20644=DIRECTION('ref_axis',(1.,0.,0.));
#20645=DIRECTION('',(0.,0.,1.));
#20646=DIRECTION('',(-1.,0.,0.));
#20647=DIRECTION('center_axis',(0.,0.,1.));
#20648=DIRECTION('ref_axis',(-1.,-2.96059473233374E-15,0.));
#20649=DIRECTION('',(0.,0.,1.));
#20650=DIRECTION('center_axis',(0.,0.,-1.));
#20651=DIRECTION('ref_axis',(-0.707106781186547,-0.707106781186548,0.));
#20652=DIRECTION('center_axis',(-1.,0.,0.));
#20653=DIRECTION('ref_axis',(0.,-1.,0.));
#20654=DIRECTION('',(0.,0.,1.));
#20655=DIRECTION('',(0.,1.,0.));
#20656=DIRECTION('center_axis',(-1.,0.,0.));
#20657=DIRECTION('ref_axis',(0.,1.,0.));
#20658=DIRECTION('center_axis',(0.,0.,1.));
#20659=DIRECTION('ref_axis',(1.,0.,0.));
#20660=DIRECTION('center_axis',(0.,0.,-1.));
#20661=DIRECTION('ref_axis',(1.,0.,0.));
#20662=DIRECTION('center_axis',(0.,0.,-1.));
#20663=DIRECTION('ref_axis',(1.,0.,0.));
#20664=DIRECTION('center_axis',(0.,0.,-1.));
#20665=DIRECTION('ref_axis',(1.,0.,0.));
#20666=DIRECTION('center_axis',(0.,-1.,0.));
#20667=DIRECTION('ref_axis',(-0.707106781186552,0.,-0.707106781186543));
#20668=DIRECTION('center_axis',(0.,-1.,0.));
#20669=DIRECTION('ref_axis',(-1.,0.,0.));
#20670=DIRECTION('',(0.,-1.,0.));
#20671=DIRECTION('center_axis',(2.96059473233373E-15,1.,0.));
#20672=DIRECTION('ref_axis',(0.,0.,-1.));
#20673=DIRECTION('center_axis',(0.,0.,1.));
#20674=DIRECTION('ref_axis',(1.,0.,0.));
#20675=DIRECTION('center_axis',(-1.,0.,0.));
#20676=DIRECTION('ref_axis',(0.,0.,-1.));
#20677=DIRECTION('center_axis',(0.,0.,1.));
#20678=DIRECTION('ref_axis',(-0.707106781186547,-0.707106781186548,0.));
#20679=DIRECTION('center_axis',(1.,0.,0.));
#20680=DIRECTION('ref_axis',(0.,-0.707106781186545,-0.70710678118655));
#20681=DIRECTION('center_axis',(-1.,0.,0.));
#20682=DIRECTION('ref_axis',(0.,0.,-1.));
#20683=DIRECTION('',(1.,0.,0.));
#20684=DIRECTION('center_axis',(0.,0.,1.));
#20685=DIRECTION('ref_axis',(1.,0.,0.));
#20686=DIRECTION('center_axis',(0.,-1.,0.));
#20687=DIRECTION('ref_axis',(0.,0.,-1.));
#20688=DIRECTION('center_axis',(0.,0.,1.));
#20689=DIRECTION('ref_axis',(0.707106781186547,-0.707106781186548,0.));
#20690=DIRECTION('center_axis',(0.,1.,0.));
#20691=DIRECTION('ref_axis',(0.707106781186548,0.,-0.707106781186548));
#20692=DIRECTION('center_axis',(-2.96059473233374E-15,-1.,0.));
#20693=DIRECTION('ref_axis',(0.,0.,-1.));
#20694=DIRECTION('',(0.,-1.,0.));
#20695=DIRECTION('',(0.,1.,0.));
#20696=DIRECTION('center_axis',(0.,0.,1.));
#20697=DIRECTION('ref_axis',(1.,0.,0.));
#20698=DIRECTION('center_axis',(1.,0.,0.));
#20699=DIRECTION('ref_axis',(0.,0.,-1.));
#20700=DIRECTION('center_axis',(0.,0.,-1.));
#20701=DIRECTION('ref_axis',(0.707106781186547,0.707106781186548,0.));
#20702=DIRECTION('center_axis',(0.,0.,1.));
#20703=DIRECTION('ref_axis',(0.707106781186547,0.707106781186548,0.));
#20704=DIRECTION('center_axis',(-1.,0.,0.));
#20705=DIRECTION('ref_axis',(0.,0.707106781186545,-0.70710678118655));
#20706=DIRECTION('center_axis',(1.,0.,0.));
#20707=DIRECTION('ref_axis',(0.,0.,-1.));
#20708=DIRECTION('',(1.,0.,0.));
#20709=DIRECTION('',(-1.,0.,0.));
#20710=DIRECTION('center_axis',(0.,0.,1.));
#20711=DIRECTION('ref_axis',(1.,0.,0.));
#20712=DIRECTION('center_axis',(0.,0.,-1.));
#20713=DIRECTION('ref_axis',(-0.707106781186547,0.707106781186548,0.));
#20714=DIRECTION('center_axis',(0.,0.,1.));
#20715=DIRECTION('ref_axis',(-0.707106781186547,0.707106781186548,0.));
#20716=DIRECTION('center_axis',(0.,0.,1.));
#20717=DIRECTION('ref_axis',(1.,0.,0.));
#20718=DIRECTION('',(0.,0.,1.));
#20719=DIRECTION('',(0.,0.,1.));
#20720=DIRECTION('center_axis',(0.,1.,0.));
#20721=DIRECTION('ref_axis',(-1.,0.,0.));
#20722=DIRECTION('',(0.,0.,1.));
#20723=DIRECTION('center_axis',(0.,0.,1.));
#20724=DIRECTION('ref_axis',(-1.48029736616687E-15,1.,0.));
#20725=DIRECTION('center_axis',(0.,0.,1.));
#20726=DIRECTION('ref_axis',(1.,0.,0.));
#20727=DIRECTION('center_axis',(0.,0.,1.));
#20728=DIRECTION('ref_axis',(1.,0.,0.));
#20729=DIRECTION('center_axis',(0.,0.,1.));
#20730=DIRECTION('ref_axis',(1.,0.,0.));
#20731=DIRECTION('center_axis',(0.754605522163505,7.28504717578445E-17,
0.656178714924787));
#20732=DIRECTION('ref_axis',(-0.656178714924787,0.,0.754605522163505));
#20733=DIRECTION('center_axis',(0.754605522163505,7.28504717578445E-17,
0.656178714924787));
#20734=DIRECTION('ref_axis',(-0.656178714924787,0.,0.754605522163505));
#20735=DIRECTION('center_axis',(-0.754605522163505,-7.28504717578445E-17,
0.656178714924787));
#20736=DIRECTION('ref_axis',(0.656178714924787,0.,0.754605522163505));
#20737=DIRECTION('center_axis',(0.754605522163505,7.28504717578445E-17,
0.656178714924787));
#20738=DIRECTION('ref_axis',(-0.656178714924787,0.,0.754605522163505));
#20739=DIRECTION('center_axis',(0.754605522163505,7.28504717578445E-17,
0.656178714924787));
#20740=DIRECTION('ref_axis',(-0.656178714924787,0.,0.754605522163505));
#20741=DIRECTION('center_axis',(-0.754605522163505,-7.28504717578445E-17,
0.656178714924787));
#20742=DIRECTION('ref_axis',(0.656178714924787,0.,0.754605522163505));
#20743=DIRECTION('center_axis',(0.,0.,-1.));
#20744=DIRECTION('ref_axis',(1.,0.,0.));
#20745=DIRECTION('',(0.,0.,-1.));
#20746=DIRECTION('center_axis',(0.,0.,-1.));
#20747=DIRECTION('ref_axis',(1.,0.,0.));
#20748=DIRECTION('',(0.,0.,-1.));
#20749=DIRECTION('center_axis',(0.,0.,-1.));
#20750=DIRECTION('ref_axis',(1.,0.,0.));
#20751=DIRECTION('',(0.,0.,-1.));
#20752=DIRECTION('center_axis',(0.,0.,-1.));
#20753=DIRECTION('ref_axis',(1.,0.,0.));
#20754=DIRECTION('',(0.,0.,-1.));
#20755=DIRECTION('center_axis',(0.,0.,-1.));
#20756=DIRECTION('ref_axis',(1.,0.,0.));
#20757=DIRECTION('',(0.,0.,-1.));
#20758=DIRECTION('center_axis',(0.,0.,-1.));
#20759=DIRECTION('ref_axis',(1.,0.,0.));
#20760=DIRECTION('',(0.,0.,-1.));
#20761=DIRECTION('center_axis',(1.,0.,0.));
#20762=DIRECTION('ref_axis',(0.,1.,0.));
#20763=DIRECTION('',(1.,0.,0.));
#20764=DIRECTION('center_axis',(-1.,0.,0.));
#20765=DIRECTION('ref_axis',(0.,0.,1.));
#20766=DIRECTION('center_axis',(1.,0.,0.));
#20767=DIRECTION('ref_axis',(0.,1.,0.));
#20768=DIRECTION('center_axis',(1.,0.,0.));
#20769=DIRECTION('ref_axis',(0.,1.,0.));
#20770=DIRECTION('center_axis',(1.,0.,0.));
#20771=DIRECTION('ref_axis',(0.,1.,0.));
#20772=DIRECTION('',(-1.,0.,0.));
#20773=DIRECTION('center_axis',(1.,0.,0.));
#20774=DIRECTION('ref_axis',(0.,1.,0.));
#20775=DIRECTION('center_axis',(1.,0.,0.));
#20776=DIRECTION('ref_axis',(0.,1.,0.));
#20777=DIRECTION('center_axis',(1.,0.,0.));
#20778=DIRECTION('ref_axis',(0.,1.,0.));
#20779=DIRECTION('',(-1.,0.,0.));
#20780=DIRECTION('center_axis',(1.,0.,0.));
#20781=DIRECTION('ref_axis',(0.,1.,0.));
#20782=DIRECTION('',(-1.,0.,0.));
#33502=CARTESIAN_POINT('',(0.,0.,0.));
#33503=CARTESIAN_POINT('Origin',(-79.75,0.,0.));
#33504=CARTESIAN_POINT('',(-80.,10.5,-1.28587913910472E-15));
#33505=CARTESIAN_POINT('Origin',(-80.,0.,0.));
#33506=CARTESIAN_POINT('',(-79.5,10.,1.22464679914735E-15));
#33507=CARTESIAN_POINT('',(-79.75,10.25,-1.25526296912604E-15));
#33508=CARTESIAN_POINT('',(-79.5,-10.,-1.22464679914735E-15));
#33509=CARTESIAN_POINT('Origin',(-79.5,0.,0.));
#33510=CARTESIAN_POINT('Origin',(-79.5,0.,0.));
#33511=CARTESIAN_POINT('Origin',(-80.,10.,0.));
#33512=CARTESIAN_POINT('',(-80.,-12.05,-1.47569939297256E-15));
#33513=CARTESIAN_POINT('Origin',(-80.,0.,0.));
#33514=CARTESIAN_POINT('Origin',(14.,0.,0.));
#33515=CARTESIAN_POINT('',(-61.,-10.,0.));
#33516=CARTESIAN_POINT('',(14.,-10.,-1.22464679914735E-15));
#33517=CARTESIAN_POINT('',(61.,-10.,0.));
#33518=CARTESIAN_POINT('',(14.,-10.,-1.22464679914735E-15));
#33519=CARTESIAN_POINT('',(108.,-10.,-1.22464679914735E-15));
#33520=CARTESIAN_POINT('',(14.,-10.,-1.22464679914735E-15));
#33521=CARTESIAN_POINT('Origin',(108.,0.,0.));
#33522=CARTESIAN_POINT('',(61.,10.,0.));
#33523=CARTESIAN_POINT('Origin',(61.,0.,0.));
#33524=CARTESIAN_POINT('Origin',(61.,0.,0.));
#33525=CARTESIAN_POINT('',(-61.,10.,0.));
#33526=CARTESIAN_POINT('Origin',(-61.,0.,0.));
#33527=CARTESIAN_POINT('Origin',(-61.,0.,0.));
#33528=CARTESIAN_POINT('Origin',(125.75,0.,0.));
#33529=CARTESIAN_POINT('',(126.,-11.05,-1.35323471305783E-15));
#33530=CARTESIAN_POINT('Origin',(126.,0.,0.));
#33531=CARTESIAN_POINT('',(125.5,-10.55,1.29200237310046E-15));
#33532=CARTESIAN_POINT('',(125.75,-10.8,-1.32261854307914E-15));
#33533=CARTESIAN_POINT('Origin',(125.5,0.,0.));
#33534=CARTESIAN_POINT('Origin',(126.,0.,0.));
#33535=CARTESIAN_POINT('',(126.,-15.5,4.11864858792871E-15));
#33536=CARTESIAN_POINT('Origin',(126.,0.,0.));
#33537=CARTESIAN_POINT('Origin',(117.05,0.,0.));
#33538=CARTESIAN_POINT('',(108.,-10.55,-1.29200237310046E-15));
#33539=CARTESIAN_POINT('Origin',(108.,0.,0.));
#33540=CARTESIAN_POINT('',(117.05,-10.55,-1.29200237310046E-15));
#33541=CARTESIAN_POINT('Origin',(124.5,0.,0.));
#33542=CARTESIAN_POINT('',(124.5,-17.,3.53428366433714E-16));
#33543=CARTESIAN_POINT('Origin',(124.5,0.,0.));
#33544=CARTESIAN_POINT('Origin',(124.5,-15.5,3.22243510571916E-16));
#33545=CARTESIAN_POINT('Origin',(112.75,0.,0.));
#33546=CARTESIAN_POINT('',(101.5,-17.,-2.0818995585505E-15));
#33547=CARTESIAN_POINT('',(112.75,-17.,-2.0818995585505E-15));
#33548=CARTESIAN_POINT('',(101.5,-2.0818995585505E-15,17.));
#33549=CARTESIAN_POINT('Origin',(101.5,0.,0.));
#33550=CARTESIAN_POINT('Origin',(101.5,0.,0.));
#33551=CARTESIAN_POINT('Origin',(101.5,0.,0.));
#33552=CARTESIAN_POINT('',(100.,-1.8982025386784E-15,15.5));
#33553=CARTESIAN_POINT('Origin',(101.5,-1.8982025386784E-15,15.5));
#33554=CARTESIAN_POINT('Origin',(100.,0.,0.));
#33555=CARTESIAN_POINT('Origin',(100.,17.,0.));
#33556=CARTESIAN_POINT('',(100.,-14.,-1.71450551880629E-15));
#33557=CARTESIAN_POINT('Origin',(100.,0.,0.));
#33558=CARTESIAN_POINT('Origin',(-81.5,0.,0.));
#33559=CARTESIAN_POINT('',(-80.,-1.8982025386784E-15,15.5));
#33560=CARTESIAN_POINT('Origin',(-80.,0.,0.));
#33561=CARTESIAN_POINT('',(-81.5,-2.0818995585505E-15,17.));
#33562=CARTESIAN_POINT('Origin',(-81.5,-1.8982025386784E-15,15.5));
#33563=CARTESIAN_POINT('',(-81.5,-17.,-2.0818995585505E-15));
#33564=CARTESIAN_POINT('Origin',(-81.5,0.,0.));
#33565=CARTESIAN_POINT('Origin',(-81.5,0.,0.));
#33566=CARTESIAN_POINT('Origin',(-84.75,0.,0.));
#33567=CARTESIAN_POINT('',(-88.5,-17.,0.));
#33568=CARTESIAN_POINT('',(-84.75,-17.,-2.0818995585505E-15));
#33569=CARTESIAN_POINT('Origin',(-88.5,0.,0.));
#33570=CARTESIAN_POINT('Origin',(-80.,14.,0.));
#33571=CARTESIAN_POINT('',(-80.,-14.,-1.71450551880629E-15));
#33572=CARTESIAN_POINT('Origin',(-80.,0.,0.));
#33573=CARTESIAN_POINT('Origin',(-88.5,0.,0.));
#33574=CARTESIAN_POINT('',(-90.,-15.5,-3.79640507735679E-15));
#33575=CARTESIAN_POINT('Origin',(-88.5,-15.5,0.));
#33576=CARTESIAN_POINT('Origin',(-90.,0.,0.));
#33577=CARTESIAN_POINT('Origin',(-90.,16.5,0.));
#33578=CARTESIAN_POINT('',(-90.,-12.05,-1.47569939297256E-15));
#33579=CARTESIAN_POINT('Origin',(-90.,0.,0.));
#33580=CARTESIAN_POINT('Origin',(-77.5,13.5,16.5));
#33581=CARTESIAN_POINT('',(-77.5,27.,18.));
#33582=CARTESIAN_POINT('',(-79.,27.,16.5));
#33583=CARTESIAN_POINT('Origin',(-77.5,27.,16.5));
#33584=CARTESIAN_POINT('',(-79.,-27.,16.5));
#33585=CARTESIAN_POINT('',(-79.,13.5,16.5));
#33586=CARTESIAN_POINT('',(-77.5,-27.,18.));
#33587=CARTESIAN_POINT('Origin',(-77.5,-27.,16.5));
#33588=CARTESIAN_POINT('',(-77.5,13.5,18.));
#33589=CARTESIAN_POINT('Origin',(-73.,-27.,16.5));
#33590=CARTESIAN_POINT('',(-73.,-33.,16.5));
#33591=CARTESIAN_POINT('',(-73.,-31.5,18.));
#33592=CARTESIAN_POINT('Origin',(-73.,-31.5,16.5));
#33593=CARTESIAN_POINT('Origin',(-73.,-27.,18.));
#33594=CARTESIAN_POINT('Origin',(-73.,-27.,16.5));
#33595=CARTESIAN_POINT('Origin',(-67.,-31.5,16.5));
#33596=CARTESIAN_POINT('',(-49.,-33.,16.5));
#33597=CARTESIAN_POINT('',(-49.,-31.5,18.));
#33598=CARTESIAN_POINT('Origin',(-49.,-31.5,16.5));
#33599=CARTESIAN_POINT('',(-67.,-31.5,18.));
#33600=CARTESIAN_POINT('',(-67.,-33.,16.5));
#33601=CARTESIAN_POINT('Origin',(-49.,-27.,16.5));
#33602=CARTESIAN_POINT('',(-43.,-27.,16.5));
#33603=CARTESIAN_POINT('',(-44.5,-27.,18.));
#33604=CARTESIAN_POINT('Origin',(-44.5,-27.,16.5));
#33605=CARTESIAN_POINT('Origin',(-49.,-27.,18.));
#33606=CARTESIAN_POINT('Origin',(-49.,-27.,16.5));
#33607=CARTESIAN_POINT('Origin',(-44.5,-13.5,16.5));
#33608=CARTESIAN_POINT('',(-43.,27.,16.5));
#33609=CARTESIAN_POINT('',(-44.5,27.,18.));
#33610=CARTESIAN_POINT('Origin',(-44.5,27.,16.5));
#33611=CARTESIAN_POINT('',(-44.5,-13.5,18.));
#33612=CARTESIAN_POINT('',(-43.,-13.5,16.5));
#33613=CARTESIAN_POINT('Origin',(-49.,27.,16.5));
#33614=CARTESIAN_POINT('',(-49.,33.,16.5));
#33615=CARTESIAN_POINT('',(-49.,31.5,18.));
#33616=CARTESIAN_POINT('Origin',(-49.,31.5,16.5));
#33617=CARTESIAN_POINT('Origin',(-49.,27.,18.));
#33618=CARTESIAN_POINT('Origin',(-49.,27.,16.5));
#33619=CARTESIAN_POINT('Origin',(-55.,31.5,16.5));
#33620=CARTESIAN_POINT('',(-73.,33.,16.5));
#33621=CARTESIAN_POINT('',(-73.,31.5,18.));
#33622=CARTESIAN_POINT('Origin',(-73.,31.5,16.5));
#33623=CARTESIAN_POINT('',(-55.,31.5,18.));
#33624=CARTESIAN_POINT('',(-55.,33.,16.5));
#33625=CARTESIAN_POINT('Origin',(-73.,27.,16.5));
#33626=CARTESIAN_POINT('Origin',(-73.,27.,18.));
#33627=CARTESIAN_POINT('Origin',(-73.,27.,16.5));
#33628=CARTESIAN_POINT('Origin',(-49.,-27.,-24.));
#33629=CARTESIAN_POINT('',(-49.,-33.,-22.5));
#33630=CARTESIAN_POINT('',(-49.,-33.,-24.));
#33631=CARTESIAN_POINT('',(-43.,-27.,-22.5));
#33632=CARTESIAN_POINT('Origin',(-49.,-27.,-22.5));
#33633=CARTESIAN_POINT('',(-43.,-27.,-24.));
#33634=CARTESIAN_POINT('Origin',(-73.,-33.,-24.));
#33635=CARTESIAN_POINT('',(-73.,-33.,-22.5));
#33636=CARTESIAN_POINT('',(-73.,-33.,-24.));
#33637=CARTESIAN_POINT('',(-67.,-33.,-22.5));
#33638=CARTESIAN_POINT('Origin',(-73.,-27.,-24.));
#33639=CARTESIAN_POINT('',(-79.,-27.,-22.5));
#33640=CARTESIAN_POINT('',(-79.,-27.,-24.));
#33641=CARTESIAN_POINT('Origin',(-73.,-27.,-22.5));
#33642=CARTESIAN_POINT('Origin',(-79.,27.,-24.));
#33643=CARTESIAN_POINT('',(-79.,27.,-22.5));
#33644=CARTESIAN_POINT('',(-79.,27.,-24.));
#33645=CARTESIAN_POINT('',(-79.,13.5,-22.5));
#33646=CARTESIAN_POINT('',(-79.,-14.,1.71450551880629E-15));
#33647=CARTESIAN_POINT('Origin',(-79.,0.,0.));
#33648=CARTESIAN_POINT('Origin',(-61.,0.,18.));
#33649=CARTESIAN_POINT('',(-71.,-1.22464679914735E-15,18.));
#33650=CARTESIAN_POINT('Origin',(-61.,0.,18.));
#33651=CARTESIAN_POINT('',(-65.5,-25.,18.));
#33652=CARTESIAN_POINT('Origin',(-61.,-25.,18.));
#33653=CARTESIAN_POINT('',(-65.5,25.,18.));
#33654=CARTESIAN_POINT('Origin',(-61.,25.,18.));
#33655=CARTESIAN_POINT('Origin',(-77.5,13.5,-22.5));
#33656=CARTESIAN_POINT('',(-77.5,27.,-24.));
#33657=CARTESIAN_POINT('Origin',(-77.5,27.,-22.5));
#33658=CARTESIAN_POINT('',(-77.5,-27.,-24.));
#33659=CARTESIAN_POINT('',(-77.5,13.5,-24.));
#33660=CARTESIAN_POINT('Origin',(-77.5,-27.,-22.5));
#33661=CARTESIAN_POINT('Origin',(-73.,-27.,-22.5));
#33662=CARTESIAN_POINT('',(-73.,-31.5,-24.));
#33663=CARTESIAN_POINT('Origin',(-73.,-31.5,-22.5));
#33664=CARTESIAN_POINT('Origin',(-73.,-27.,-24.));
#33665=CARTESIAN_POINT('Origin',(-67.,-31.5,-22.5));
#33666=CARTESIAN_POINT('',(-49.,-31.5,-24.));
#33667=CARTESIAN_POINT('Origin',(-49.,-31.5,-22.5));
#33668=CARTESIAN_POINT('',(-67.,-31.5,-24.));
#33669=CARTESIAN_POINT('Origin',(-49.,-27.,-22.5));
#33670=CARTESIAN_POINT('',(-44.5,-27.,-24.));
#33671=CARTESIAN_POINT('Origin',(-44.5,-27.,-22.5));
#33672=CARTESIAN_POINT('Origin',(-49.,-27.,-24.));
#33673=CARTESIAN_POINT('Origin',(-44.5,-13.5,-22.5));
#33674=CARTESIAN_POINT('',(-44.5,27.,-24.));
#33675=CARTESIAN_POINT('',(-43.,27.,-22.5));
#33676=CARTESIAN_POINT('Origin',(-44.5,27.,-22.5));
#33677=CARTESIAN_POINT('',(-43.,-13.5,-22.5));
#33678=CARTESIAN_POINT('',(-44.5,-13.5,-24.));
#33679=CARTESIAN_POINT('Origin',(-49.,27.,-22.5));
#33680=CARTESIAN_POINT('',(-49.,31.5,-24.));
#33681=CARTESIAN_POINT('',(-49.,33.,-22.5));
#33682=CARTESIAN_POINT('Origin',(-49.,31.5,-22.5));
#33683=CARTESIAN_POINT('Origin',(-49.,27.,-22.5));
#33684=CARTESIAN_POINT('Origin',(-49.,27.,-24.));
#33685=CARTESIAN_POINT('Origin',(-55.,31.5,-22.5));
#33686=CARTESIAN_POINT('',(-73.,31.5,-24.));
#33687=CARTESIAN_POINT('',(-73.,33.,-22.5));
#33688=CARTESIAN_POINT('Origin',(-73.,31.5,-22.5));
#33689=CARTESIAN_POINT('',(-55.,33.,-22.5));
#33690=CARTESIAN_POINT('',(-55.,31.5,-24.));
#33691=CARTESIAN_POINT('Origin',(-73.,27.,-22.5));
#33692=CARTESIAN_POINT('Origin',(-73.,27.,-22.5));
#33693=CARTESIAN_POINT('Origin',(-73.,27.,-24.));
#33694=CARTESIAN_POINT('Origin',(-49.,27.,-24.));
#33695=CARTESIAN_POINT('',(-43.,27.,-24.));
#33696=CARTESIAN_POINT('',(-49.,33.,-24.));
#33697=CARTESIAN_POINT('Origin',(-49.,33.,-24.));
#33698=CARTESIAN_POINT('',(-73.,33.,-24.));
#33699=CARTESIAN_POINT('Origin',(-73.,27.,-24.));
#33700=CARTESIAN_POINT('Origin',(-61.,0.,-24.));
#33701=CARTESIAN_POINT('',(-65.5,-25.,-24.));
#33702=CARTESIAN_POINT('Origin',(-61.,-25.,-24.));
#33703=CARTESIAN_POINT('',(-65.5,25.,-24.));
#33704=CARTESIAN_POINT('Origin',(-61.,25.,-24.));
#33705=CARTESIAN_POINT('Origin',(44.5,13.5,16.5));
#33706=CARTESIAN_POINT('',(44.5,27.,18.));
#33707=CARTESIAN_POINT('',(43.,27.,16.5));
#33708=CARTESIAN_POINT('Origin',(44.5,27.,16.5));
#33709=CARTESIAN_POINT('',(43.,-27.,16.5));
#33710=CARTESIAN_POINT('',(43.,13.5,16.5));
#33711=CARTESIAN_POINT('',(44.5,-27.,18.));
#33712=CARTESIAN_POINT('Origin',(44.5,-27.,16.5));
#33713=CARTESIAN_POINT('',(44.5,13.5,18.));
#33714=CARTESIAN_POINT('Origin',(49.,-27.,16.5));
#33715=CARTESIAN_POINT('',(49.,-33.,16.5));
#33716=CARTESIAN_POINT('',(49.,-31.5,18.));
#33717=CARTESIAN_POINT('Origin',(49.,-31.5,16.5));
#33718=CARTESIAN_POINT('Origin',(49.,-27.,18.));
#33719=CARTESIAN_POINT('Origin',(49.,-27.,16.5));
#33720=CARTESIAN_POINT('Origin',(55.,-31.5,16.5));
#33721=CARTESIAN_POINT('',(73.,-33.,16.5));
#33722=CARTESIAN_POINT('',(73.,-31.5,18.));
#33723=CARTESIAN_POINT('Origin',(73.,-31.5,16.5));
#33724=CARTESIAN_POINT('',(55.,-31.5,18.));
#33725=CARTESIAN_POINT('',(55.,-33.,16.5));
#33726=CARTESIAN_POINT('Origin',(73.,-27.,16.5));
#33727=CARTESIAN_POINT('',(79.,-27.,16.5));
#33728=CARTESIAN_POINT('',(77.5,-27.,18.));
#33729=CARTESIAN_POINT('Origin',(77.5,-27.,16.5));
#33730=CARTESIAN_POINT('Origin',(73.,-27.,18.));
#33731=CARTESIAN_POINT('Origin',(73.,-27.,16.5));
#33732=CARTESIAN_POINT('Origin',(77.5,-13.5,16.5));
#33733=CARTESIAN_POINT('',(79.,27.,16.5));
#33734=CARTESIAN_POINT('',(77.5,27.,18.));
#33735=CARTESIAN_POINT('Origin',(77.5,27.,16.5));
#33736=CARTESIAN_POINT('',(77.5,-13.5,18.));
#33737=CARTESIAN_POINT('',(79.,-13.5,16.5));
#33738=CARTESIAN_POINT('Origin',(73.,27.,16.5));
#33739=CARTESIAN_POINT('',(73.,33.,16.5));
#33740=CARTESIAN_POINT('',(73.,31.5,18.));
#33741=CARTESIAN_POINT('Origin',(73.,31.5,16.5));
#33742=CARTESIAN_POINT('Origin',(73.,27.,18.));
#33743=CARTESIAN_POINT('Origin',(73.,27.,16.5));
#33744=CARTESIAN_POINT('Origin',(67.,31.5,16.5));
#33745=CARTESIAN_POINT('',(49.,33.,16.5));
#33746=CARTESIAN_POINT('',(49.,31.5,18.));
#33747=CARTESIAN_POINT('Origin',(49.,31.5,16.5));
#33748=CARTESIAN_POINT('',(67.,31.5,18.));
#33749=CARTESIAN_POINT('',(67.,33.,16.5));
#33750=CARTESIAN_POINT('Origin',(49.,27.,16.5));
#33751=CARTESIAN_POINT('Origin',(49.,27.,18.));
#33752=CARTESIAN_POINT('Origin',(49.,27.,16.5));
#33753=CARTESIAN_POINT('Origin',(73.,-27.,-24.));
#33754=CARTESIAN_POINT('',(73.,-33.,-22.5));
#33755=CARTESIAN_POINT('',(73.,-33.,-24.));
#33756=CARTESIAN_POINT('',(79.,-27.,-22.5));
#33757=CARTESIAN_POINT('Origin',(73.,-27.,-22.5));
#33758=CARTESIAN_POINT('',(79.,-27.,-24.));
#33759=CARTESIAN_POINT('Origin',(49.,-33.,-24.));
#33760=CARTESIAN_POINT('',(49.,-33.,-22.5));
#33761=CARTESIAN_POINT('',(49.,-33.,-24.));
#33762=CARTESIAN_POINT('',(55.,-33.,-22.5));
#33763=CARTESIAN_POINT('Origin',(49.,-27.,-24.));
#33764=CARTESIAN_POINT('',(43.,-27.,-22.5));
#33765=CARTESIAN_POINT('',(43.,-27.,-24.));
#33766=CARTESIAN_POINT('Origin',(49.,-27.,-22.5));
#33767=CARTESIAN_POINT('Origin',(43.,27.,-24.));
#33768=CARTESIAN_POINT('',(43.,27.,-22.5));
#33769=CARTESIAN_POINT('',(43.,27.,-24.));
#33770=CARTESIAN_POINT('',(43.,13.5,-22.5));
#33771=CARTESIAN_POINT('',(43.,-14.,1.71450551880629E-15));
#33772=CARTESIAN_POINT('Origin',(43.,0.,0.));
#33773=CARTESIAN_POINT('Origin',(61.,0.,18.));
#33774=CARTESIAN_POINT('',(51.,-1.22464679914735E-15,18.));
#33775=CARTESIAN_POINT('Origin',(61.,0.,18.));
#33776=CARTESIAN_POINT('',(56.5,25.,18.));
#33777=CARTESIAN_POINT('Origin',(61.,25.,18.));
#33778=CARTESIAN_POINT('',(56.5,-25.,18.));
#33779=CARTESIAN_POINT('Origin',(61.,-25.,18.));
#33780=CARTESIAN_POINT('Origin',(44.5,13.5,-22.5));
#33781=CARTESIAN_POINT('',(44.5,27.,-24.));
#33782=CARTESIAN_POINT('Origin',(44.5,27.,-22.5));
#33783=CARTESIAN_POINT('',(44.5,-27.,-24.));
#33784=CARTESIAN_POINT('',(44.5,13.5,-24.));
#33785=CARTESIAN_POINT('Origin',(44.5,-27.,-22.5));
#33786=CARTESIAN_POINT('Origin',(49.,-27.,-22.5));
#33787=CARTESIAN_POINT('',(49.,-31.5,-24.));
#33788=CARTESIAN_POINT('Origin',(49.,-31.5,-22.5));
#33789=CARTESIAN_POINT('Origin',(49.,-27.,-24.));
#33790=CARTESIAN_POINT('Origin',(55.,-31.5,-22.5));
#33791=CARTESIAN_POINT('',(73.,-31.5,-24.));
#33792=CARTESIAN_POINT('Origin',(73.,-31.5,-22.5));
#33793=CARTESIAN_POINT('',(55.,-31.5,-24.));
#33794=CARTESIAN_POINT('Origin',(73.,-27.,-22.5));
#33795=CARTESIAN_POINT('',(77.5,-27.,-24.));
#33796=CARTESIAN_POINT('Origin',(77.5,-27.,-22.5));
#33797=CARTESIAN_POINT('Origin',(73.,-27.,-24.));
#33798=CARTESIAN_POINT('Origin',(77.5,-13.5,-22.5));
#33799=CARTESIAN_POINT('',(77.5,27.,-24.));
#33800=CARTESIAN_POINT('',(79.,27.,-22.5));
#33801=CARTESIAN_POINT('Origin',(77.5,27.,-22.5));
#33802=CARTESIAN_POINT('',(79.,-13.5,-22.5));
#33803=CARTESIAN_POINT('',(77.5,-13.5,-24.));
#33804=CARTESIAN_POINT('Origin',(73.,27.,-22.5));
#33805=CARTESIAN_POINT('',(73.,31.5,-24.));
#33806=CARTESIAN_POINT('',(73.,33.,-22.5));
#33807=CARTESIAN_POINT('Origin',(73.,31.5,-22.5));
#33808=CARTESIAN_POINT('Origin',(73.,27.,-22.5));
#33809=CARTESIAN_POINT('Origin',(73.,27.,-24.));
#33810=CARTESIAN_POINT('Origin',(67.,31.5,-22.5));
#33811=CARTESIAN_POINT('',(49.,31.5,-24.));
#33812=CARTESIAN_POINT('',(49.,33.,-22.5));
#33813=CARTESIAN_POINT('Origin',(49.,31.5,-22.5));
#33814=CARTESIAN_POINT('',(67.,33.,-22.5));
#33815=CARTESIAN_POINT('',(67.,31.5,-24.));
#33816=CARTESIAN_POINT('Origin',(49.,27.,-22.5));
#33817=CARTESIAN_POINT('Origin',(49.,27.,-22.5));
#33818=CARTESIAN_POINT('Origin',(49.,27.,-24.));
#33819=CARTESIAN_POINT('Origin',(73.,27.,-24.));
#33820=CARTESIAN_POINT('',(79.,27.,-24.));
#33821=CARTESIAN_POINT('',(73.,33.,-24.));
#33822=CARTESIAN_POINT('Origin',(73.,33.,-24.));
#33823=CARTESIAN_POINT('',(49.,33.,-24.));
#33824=CARTESIAN_POINT('Origin',(49.,27.,-24.));
#33825=CARTESIAN_POINT('Origin',(61.,0.,-24.));
#33826=CARTESIAN_POINT('',(56.5,25.,-24.));
#33827=CARTESIAN_POINT('Origin',(61.,25.,-24.));
#33828=CARTESIAN_POINT('',(56.5,-25.,-24.));
#33829=CARTESIAN_POINT('Origin',(61.,-25.,-24.));
#33830=CARTESIAN_POINT('Ctrl Pts',(61.,10.,0.));
#33831=CARTESIAN_POINT('Ctrl Pts',(59.5040034982906,10.,1.72039597696584));
#33832=CARTESIAN_POINT('Ctrl Pts',(56.5121809687138,9.31827600185967,5.16099188597912));
#33833=CARTESIAN_POINT('Ctrl Pts',(52.9151698102436,6.44751899352647,9.29755471821987));
#33834=CARTESIAN_POINT('Ctrl Pts',(50.916118401284,2.30148284591066,11.5964638385234));
#33835=CARTESIAN_POINT('Ctrl Pts',(50.9184096402541,-2.30110422892933,11.5938289137078));
#33836=CARTESIAN_POINT('Ctrl Pts',(52.9132003149412,-6.44872389556736,9.29981963781766));
#33837=CARTESIAN_POINT('Ctrl Pts',(56.5134223825492,-9.3173037934771,5.15956426006841));
#33838=CARTESIAN_POINT('Ctrl Pts',(59.5040034982906,-10.,1.72039597696584));
#33839=CARTESIAN_POINT('Ctrl Pts',(61.,-10.,0.));
#33840=CARTESIAN_POINT('Ctrl Pts',(61.,10.,0.));
#33841=CARTESIAN_POINT('Ctrl Pts',(59.4612607410989,10.,1.67765321977414));
#33842=CARTESIAN_POINT('Ctrl Pts',(56.3852895451264,9.2787466754377,5.03147281006447));
#33843=CARTESIAN_POINT('Ctrl Pts',(52.7787910927581,6.28233675146603,9.01828223151668));
#33844=CARTESIAN_POINT('Ctrl Pts',(50.9218563946624,2.16780125001729,11.1411198281225));
#33845=CARTESIAN_POINT('Ctrl Pts',(50.921935151735,-2.16957611933213,11.139875359174));
#33846=CARTESIAN_POINT('Ctrl Pts',(52.7749511431933,-6.28255214648714,9.02170832410809));
#33847=CARTESIAN_POINT('Ctrl Pts',(56.3865568068429,-9.27716494796019,5.03035580652707));
#33848=CARTESIAN_POINT('Ctrl Pts',(59.4612607410989,-10.,1.67765321977414));
#33849=CARTESIAN_POINT('Ctrl Pts',(61.,-10.,-1.16633028490224E-16));
#33850=CARTESIAN_POINT('Ctrl Pts',(61.,10.,0.));
#33851=CARTESIAN_POINT('Ctrl Pts',(59.3864609160134,10.,1.60285339468867));
#33852=CARTESIAN_POINT('Ctrl Pts',(56.1634454725933,9.24997499276094,4.8044724705041));
#33853=CARTESIAN_POINT('Ctrl Pts',(52.4020469154053,6.14806419752617,8.52856750953951));
#33854=CARTESIAN_POINT('Ctrl Pts',(50.5404578733979,2.04963586749967,10.355517733166));
#33855=CARTESIAN_POINT('Ctrl Pts',(50.540659846251,-2.05249740360806,10.3555567579218));
#33856=CARTESIAN_POINT('Ctrl Pts',(52.3971494142207,-6.14820999431346,8.53360127461872));
#33857=CARTESIAN_POINT('Ctrl Pts',(56.163818037358,-9.24763407888523,4.80405041789639));
#33858=CARTESIAN_POINT('Ctrl Pts',(59.3864609160134,-10.,1.60285339468867));
#33859=CARTESIAN_POINT('Ctrl Pts',(61.,-10.,-3.20740828348117E-16));
#33860=CARTESIAN_POINT('Ctrl Pts',(61.,10.,0.));
#33861=CARTESIAN_POINT('Ctrl Pts',(59.3116610909279,10.,1.5280535696032));
#33862=CARTESIAN_POINT('Ctrl Pts',(55.9363931602234,9.28829710822045,4.58270974350988));
#33863=CARTESIAN_POINT('Ctrl Pts',(51.9123266113155,6.32379422406357,8.1866464187036));
#33864=CARTESIAN_POINT('Ctrl Pts',(49.7441230249571,2.20237919885278,10.0805955452152));
#33865=CARTESIAN_POINT('Ctrl Pts',(49.7460827491046,-2.20331916195195,10.0795573075147));
#33866=CARTESIAN_POINT('Ctrl Pts',(51.9092854431927,-6.32444064491119,8.18991583103531));
#33867=CARTESIAN_POINT('Ctrl Pts',(55.9374860580148,-9.28688811871409,4.58156316448158));
#33868=CARTESIAN_POINT('Ctrl Pts',(59.3116610909279,-10.,1.5280535696032));
#33869=CARTESIAN_POINT('Ctrl Pts',(61.,-10.,-5.2484862820601E-16));
#33870=CARTESIAN_POINT('Ctrl Pts',(61.,10.,0.));
#33871=CARTESIAN_POINT('Ctrl Pts',(59.2796040230342,10.,1.49599650170942));
#33872=CARTESIAN_POINT('Ctrl Pts',(55.8390081140209,9.31827600185966,4.48781903128619));
#33873=CARTESIAN_POINT('Ctrl Pts',(51.7024452817801,6.44751899352647,8.08483018975641));
#33874=CARTESIAN_POINT('Ctrl Pts',(49.4035361614766,2.30148284591066,10.083881598716));
#33875=CARTESIAN_POINT('Ctrl Pts',(49.4061710862922,-2.30110422892933,10.0815903597459));
#33876=CARTESIAN_POINT('Ctrl Pts',(51.7001803621823,-6.44872389556736,8.08679968505884));
#33877=CARTESIAN_POINT('Ctrl Pts',(55.8404357399316,-9.3173037934771,4.48657761745079));
#33878=CARTESIAN_POINT('Ctrl Pts',(59.2796040230342,-10.,1.49599650170942));
#33879=CARTESIAN_POINT('Ctrl Pts',(61.,-10.,-6.12323399573678E-16));
#33880=CARTESIAN_POINT('',(51.,1.22464679914735E-15,11.5));
#33881=CARTESIAN_POINT('Origin',(61.,0.,-1.11022302462516E-15));
#33882=CARTESIAN_POINT('Origin',(61.,0.,-1.11022302462516E-15));
#33883=CARTESIAN_POINT('Ctrl Pts',(61.,-10.,0.));
#33884=CARTESIAN_POINT('Ctrl Pts',(62.4959965017094,-10.,1.72039597696584));
#33885=CARTESIAN_POINT('Ctrl Pts',(65.4878388575297,-9.31826228028074,5.16101468615917));
#33886=CARTESIAN_POINT('Ctrl Pts',(69.0848089584877,-6.44748693262444,9.2975303022608));
#33887=CARTESIAN_POINT('Ctrl Pts',(71.0839062596644,-2.30147560731927,11.596492198614));
#33888=CARTESIAN_POINT('Ctrl Pts',(71.0815657345164,2.3010998930418,11.5938005946939));
#33889=CARTESIAN_POINT('Ctrl Pts',(69.0868232329507,6.44874145130402,9.29984671789331));
#33890=CARTESIAN_POINT('Ctrl Pts',(65.4865746588077,9.31727427505449,5.15956085762893));
#33891=CARTESIAN_POINT('Ctrl Pts',(62.4959965017094,10.,1.72039597696584));
#33892=CARTESIAN_POINT('Ctrl Pts',(61.,10.,0.));
#33893=CARTESIAN_POINT('Ctrl Pts',(61.,-10.,-1.16633028490224E-16));
#33894=CARTESIAN_POINT('Ctrl Pts',(62.5387392589011,-10.,1.67765321977414));
#33895=CARTESIAN_POINT('Ctrl Pts',(65.6147402149094,-9.27874444858818,5.0314839646684));
#33896=CARTESIAN_POINT('Ctrl Pts',(69.2211149565067,-6.28225704725854,9.018198244725));
#33897=CARTESIAN_POINT('Ctrl Pts',(71.0780204967536,-2.16769213476844,11.1410773775261));
#33898=CARTESIAN_POINT('Ctrl Pts',(71.0779550071476,2.16958048977102,11.139828336814));
#33899=CARTESIAN_POINT('Ctrl Pts',(69.2251092841024,6.28254286828191,9.02175516699167));
#33900=CARTESIAN_POINT('Ctrl Pts',(65.6135473050458,9.277121682446,5.03041327352834));
#33901=CARTESIAN_POINT('Ctrl Pts',(62.5387392589011,10.,1.67765321977414));
#33902=CARTESIAN_POINT('Ctrl Pts',(61.,10.,0.));
#33903=CARTESIAN_POINT('Ctrl Pts',(61.,-10.,-3.20740828348117E-16));
#33904=CARTESIAN_POINT('Ctrl Pts',(62.6135390839866,-10.,1.60285339468867));
#33905=CARTESIAN_POINT('Ctrl Pts',(65.8365086336303,-9.24999260746104,4.80443145593069));
#33906=CARTESIAN_POINT('Ctrl Pts',(69.5977546769801,-6.14807857455455,8.52836701951912));
#33907=CARTESIAN_POINT('Ctrl Pts',(71.4595637706598,-2.04957572202921,10.3555252406934));
#33908=CARTESIAN_POINT('Ctrl Pts',(71.4594638033093,2.05269181819478,10.3556714380237));
#33909=CARTESIAN_POINT('Ctrl Pts',(69.6029136286413,6.14828611739566,8.53366950962115));
#33910=CARTESIAN_POINT('Ctrl Pts',(65.8362560480664,9.24757421412897,4.80413551166672));
#33911=CARTESIAN_POINT('Ctrl Pts',(62.6135390839866,10.,1.60285339468867));
#33912=CARTESIAN_POINT('Ctrl Pts',(61.,10.,0.));
#33913=CARTESIAN_POINT('Ctrl Pts',(61.,-10.,-5.2484862820601E-16));
#33914=CARTESIAN_POINT('Ctrl Pts',(62.6883389090721,-10.,1.5280535696032));
#33915=CARTESIAN_POINT('Ctrl Pts',(66.0636051991207,-9.28829063155977,4.58271947637952));
#33916=CARTESIAN_POINT('Ctrl Pts',(70.0875935962318,-6.32376606817711,8.18655899425094));
#33917=CARTESIAN_POINT('Ctrl Pts',(72.255906691879,-2.20233839346268,10.0805696428556));
#33918=CARTESIAN_POINT('Ctrl Pts',(72.2539378332695,2.20337142560397,10.0795384423798));
#33919=CARTESIAN_POINT('Ctrl Pts',(70.0907494790084,6.32446716030411,8.18995953920261));
#33920=CARTESIAN_POINT('Ctrl Pts',(66.0625288064666,9.28684508262977,4.58161014100602));
#33921=CARTESIAN_POINT('Ctrl Pts',(62.6883389090721,10.,1.5280535696032));
#33922=CARTESIAN_POINT('Ctrl Pts',(61.,10.,0.));
#33923=CARTESIAN_POINT('Ctrl Pts',(61.,-10.,-6.12323399573678E-16));
#33924=CARTESIAN_POINT('Ctrl Pts',(62.7203959769658,-10.,1.49599650170942));
#33925=CARTESIAN_POINT('Ctrl Pts',(66.1610146861591,-9.31826228028074,4.48783885752971));
#33926=CARTESIAN_POINT('Ctrl Pts',(70.2975303022608,-6.44748693262444,8.08480895848765));
#33927=CARTESIAN_POINT('Ctrl Pts',(72.596492198614,-2.30147560731927,10.0839062596644));
#33928=CARTESIAN_POINT('Ctrl Pts',(72.5938005946939,2.3010998930418,10.0815657345164));
#33929=CARTESIAN_POINT('Ctrl Pts',(70.2998467178933,6.44874145130402,8.0868232329507));
#33930=CARTESIAN_POINT('Ctrl Pts',(66.1595608576289,9.31727427505449,4.48657465880776));
#33931=CARTESIAN_POINT('Ctrl Pts',(62.7203959769658,10.,1.49599650170942));
#33932=CARTESIAN_POINT('Ctrl Pts',(61.,10.,0.));
#33933=CARTESIAN_POINT('Origin',(61.,0.,-1.11022302462516E-15));
#33934=CARTESIAN_POINT('Ctrl Pts',(-61.,10.,0.));
#33935=CARTESIAN_POINT('Ctrl Pts',(-62.4959965017094,10.,1.72039597696584));
#33936=CARTESIAN_POINT('Ctrl Pts',(-65.4878388575297,9.31826228028074,5.16101468615917));
#33937=CARTESIAN_POINT('Ctrl Pts',(-69.0848089584877,6.44748693262444,9.2975303022608));
#33938=CARTESIAN_POINT('Ctrl Pts',(-71.0839062596644,2.30147560731927,11.596492198614));
#33939=CARTESIAN_POINT('Ctrl Pts',(-71.0815657345164,-2.3010998930418,11.5938005946939));
#33940=CARTESIAN_POINT('Ctrl Pts',(-69.0868232329507,-6.44874145130402,
9.29984671789331));
#33941=CARTESIAN_POINT('Ctrl Pts',(-65.4865746588077,-9.31727427505449,
5.15956085762893));
#33942=CARTESIAN_POINT('Ctrl Pts',(-62.4959965017094,-10.,1.72039597696584));
#33943=CARTESIAN_POINT('Ctrl Pts',(-61.,-10.,0.));
#33944=CARTESIAN_POINT('Ctrl Pts',(-61.,10.,0.));
#33945=CARTESIAN_POINT('Ctrl Pts',(-62.5387392589011,10.,1.67765321977414));
#33946=CARTESIAN_POINT('Ctrl Pts',(-65.6147402149094,9.27874444858818,5.0314839646684));
#33947=CARTESIAN_POINT('Ctrl Pts',(-69.2211149565067,6.28225704725854,9.018198244725));
#33948=CARTESIAN_POINT('Ctrl Pts',(-71.0780204967536,2.16769213476844,11.1410773775261));
#33949=CARTESIAN_POINT('Ctrl Pts',(-71.0779550071476,-2.16958048977102,
11.139828336814));
#33950=CARTESIAN_POINT('Ctrl Pts',(-69.2251092841024,-6.28254286828192,
9.02175516699167));
#33951=CARTESIAN_POINT('Ctrl Pts',(-65.6135473050458,-9.277121682446,5.03041327352834));
#33952=CARTESIAN_POINT('Ctrl Pts',(-62.5387392589011,-10.,1.67765321977414));
#33953=CARTESIAN_POINT('Ctrl Pts',(-61.,-10.,-1.16633028490224E-16));
#33954=CARTESIAN_POINT('Ctrl Pts',(-61.,10.,0.));
#33955=CARTESIAN_POINT('Ctrl Pts',(-62.6135390839866,10.,1.60285339468867));
#33956=CARTESIAN_POINT('Ctrl Pts',(-65.8365086336303,9.24999260746104,4.80443145593068));
#33957=CARTESIAN_POINT('Ctrl Pts',(-69.5977546769801,6.14807857455454,8.52836701951912));
#33958=CARTESIAN_POINT('Ctrl Pts',(-71.4595637706598,2.04957572202922,10.3555252406934));
#33959=CARTESIAN_POINT('Ctrl Pts',(-71.4594638033093,-2.05269181819478,
10.3556714380237));
#33960=CARTESIAN_POINT('Ctrl Pts',(-69.6029136286413,-6.14828611739566,
8.53366950962116));
#33961=CARTESIAN_POINT('Ctrl Pts',(-65.8362560480664,-9.24757421412897,
4.80413551166671));
#33962=CARTESIAN_POINT('Ctrl Pts',(-62.6135390839866,-10.,1.60285339468867));
#33963=CARTESIAN_POINT('Ctrl Pts',(-61.,-10.,-3.20740828348117E-16));
#33964=CARTESIAN_POINT('Ctrl Pts',(-61.,10.,0.));
#33965=CARTESIAN_POINT('Ctrl Pts',(-62.6883389090721,10.,1.5280535696032));
#33966=CARTESIAN_POINT('Ctrl Pts',(-66.0636051991207,9.28829063155977,4.58271947637952));
#33967=CARTESIAN_POINT('Ctrl Pts',(-70.0875935962318,6.32376606817712,8.18655899425094));
#33968=CARTESIAN_POINT('Ctrl Pts',(-72.255906691879,2.20233839346268,10.0805696428556));
#33969=CARTESIAN_POINT('Ctrl Pts',(-72.2539378332695,-2.20337142560396,
10.0795384423798));
#33970=CARTESIAN_POINT('Ctrl Pts',(-70.0907494790084,-6.32446716030411,
8.18995953920261));
#33971=CARTESIAN_POINT('Ctrl Pts',(-66.0625288064666,-9.28684508262977,
4.58161014100602));
#33972=CARTESIAN_POINT('Ctrl Pts',(-62.6883389090721,-10.,1.5280535696032));
#33973=CARTESIAN_POINT('Ctrl Pts',(-61.,-10.,-5.2484862820601E-16));
#33974=CARTESIAN_POINT('Ctrl Pts',(-61.,10.,0.));
#33975=CARTESIAN_POINT('Ctrl Pts',(-62.7203959769658,10.,1.49599650170942));
#33976=CARTESIAN_POINT('Ctrl Pts',(-66.1610146861591,9.31826228028074,4.48783885752971));
#33977=CARTESIAN_POINT('Ctrl Pts',(-70.2975303022608,6.44748693262445,8.08480895848765));
#33978=CARTESIAN_POINT('Ctrl Pts',(-72.596492198614,2.30147560731927,10.0839062596644));
#33979=CARTESIAN_POINT('Ctrl Pts',(-72.5938005946939,-2.3010998930418,10.0815657345164));
#33980=CARTESIAN_POINT('Ctrl Pts',(-70.2998467178933,-6.44874145130402,
8.0868232329507));
#33981=CARTESIAN_POINT('Ctrl Pts',(-66.1595608576289,-9.31727427505449,
4.48657465880776));
#33982=CARTESIAN_POINT('Ctrl Pts',(-62.7203959769658,-10.,1.49599650170942));
#33983=CARTESIAN_POINT('Ctrl Pts',(-61.,-10.,-6.12323399573678E-16));
#33984=CARTESIAN_POINT('',(-71.,1.22464679914735E-15,11.5));
#33985=CARTESIAN_POINT('Origin',(-61.,0.,-1.11022302462516E-15));
#33986=CARTESIAN_POINT('Origin',(-61.,0.,-1.11022302462516E-15));
#33987=CARTESIAN_POINT('Ctrl Pts',(-61.,-10.,0.));
#33988=CARTESIAN_POINT('Ctrl Pts',(-59.5040034982906,-10.,1.72039597696584));
#33989=CARTESIAN_POINT('Ctrl Pts',(-56.5121809687138,-9.31827600185967,
5.16099188597912));
#33990=CARTESIAN_POINT('Ctrl Pts',(-52.9151698102436,-6.44751899352647,
9.29755471821987));
#33991=CARTESIAN_POINT('Ctrl Pts',(-50.916118401284,-2.30148284591066,11.5964638385234));
#33992=CARTESIAN_POINT('Ctrl Pts',(-50.9184096402541,2.30110422892933,11.5938289137078));
#33993=CARTESIAN_POINT('Ctrl Pts',(-52.9132003149412,6.44872389556736,9.29981963781766));
#33994=CARTESIAN_POINT('Ctrl Pts',(-56.5134223825492,9.3173037934771,5.15956426006841));
#33995=CARTESIAN_POINT('Ctrl Pts',(-59.5040034982906,10.,1.72039597696584));
#33996=CARTESIAN_POINT('Ctrl Pts',(-61.,10.,0.));
#33997=CARTESIAN_POINT('Ctrl Pts',(-61.,-10.,-1.16633028490224E-16));
#33998=CARTESIAN_POINT('Ctrl Pts',(-59.4612607410989,-10.,1.67765321977414));
#33999=CARTESIAN_POINT('Ctrl Pts',(-56.3852895451264,-9.27874667543771,
5.03147281006447));
#34000=CARTESIAN_POINT('Ctrl Pts',(-52.7787910927581,-6.28233675146603,
9.01828223151668));
#34001=CARTESIAN_POINT('Ctrl Pts',(-50.9218563946624,-2.16780125001729,
11.1411198281225));
#34002=CARTESIAN_POINT('Ctrl Pts',(-50.921935151735,2.16957611933213,11.139875359174));
#34003=CARTESIAN_POINT('Ctrl Pts',(-52.7749511431933,6.28255214648713,9.0217083241081));
#34004=CARTESIAN_POINT('Ctrl Pts',(-56.3865568068429,9.27716494796019,5.03035580652706));
#34005=CARTESIAN_POINT('Ctrl Pts',(-59.4612607410989,10.,1.67765321977414));
#34006=CARTESIAN_POINT('Ctrl Pts',(-61.,10.,0.));
#34007=CARTESIAN_POINT('Ctrl Pts',(-61.,-10.,-3.20740828348117E-16));
#34008=CARTESIAN_POINT('Ctrl Pts',(-59.3864609160134,-10.,1.60285339468867));
#34009=CARTESIAN_POINT('Ctrl Pts',(-56.1634454725933,-9.24997499276093,
4.80447247050411));
#34010=CARTESIAN_POINT('Ctrl Pts',(-52.4020469154053,-6.14806419752618,
8.5285675095395));
#34011=CARTESIAN_POINT('Ctrl Pts',(-50.5404578733979,-2.04963586749967,
10.355517733166));
#34012=CARTESIAN_POINT('Ctrl Pts',(-50.540659846251,2.05249740360806,10.3555567579218));
#34013=CARTESIAN_POINT('Ctrl Pts',(-52.3971494142207,6.14820999431346,8.53360127461872));
#34014=CARTESIAN_POINT('Ctrl Pts',(-56.163818037358,9.24763407888523,4.8040504178964));
#34015=CARTESIAN_POINT('Ctrl Pts',(-59.3864609160134,10.,1.60285339468867));
#34016=CARTESIAN_POINT('Ctrl Pts',(-61.,10.,0.));
#34017=CARTESIAN_POINT('Ctrl Pts',(-61.,-10.,-5.2484862820601E-16));
#34018=CARTESIAN_POINT('Ctrl Pts',(-59.3116610909279,-10.,1.5280535696032));
#34019=CARTESIAN_POINT('Ctrl Pts',(-55.9363931602234,-9.28829710822045,
4.58270974350988));
#34020=CARTESIAN_POINT('Ctrl Pts',(-51.9123266113155,-6.32379422406357,
8.1866464187036));
#34021=CARTESIAN_POINT('Ctrl Pts',(-49.7441230249571,-2.20237919885278,
10.0805955452152));
#34022=CARTESIAN_POINT('Ctrl Pts',(-49.7460827491046,2.20331916195195,10.0795573075147));
#34023=CARTESIAN_POINT('Ctrl Pts',(-51.9092854431927,6.3244406449112,8.18991583103531));
#34024=CARTESIAN_POINT('Ctrl Pts',(-55.9374860580148,9.28688811871409,4.58156316448158));
#34025=CARTESIAN_POINT('Ctrl Pts',(-59.3116610909279,10.,1.5280535696032));
#34026=CARTESIAN_POINT('Ctrl Pts',(-61.,10.,0.));
#34027=CARTESIAN_POINT('Ctrl Pts',(-61.,-10.,-6.12323399573678E-16));
#34028=CARTESIAN_POINT('Ctrl Pts',(-59.2796040230342,-10.,1.49599650170942));
#34029=CARTESIAN_POINT('Ctrl Pts',(-55.8390081140209,-9.31827600185966,
4.48781903128619));
#34030=CARTESIAN_POINT('Ctrl Pts',(-51.7024452817801,-6.44751899352647,
8.08483018975641));
#34031=CARTESIAN_POINT('Ctrl Pts',(-49.4035361614766,-2.30148284591066,
10.083881598716));
#34032=CARTESIAN_POINT('Ctrl Pts',(-49.4061710862922,2.30110422892933,10.0815903597459));
#34033=CARTESIAN_POINT('Ctrl Pts',(-51.7001803621823,6.44872389556736,8.08679968505883));
#34034=CARTESIAN_POINT('Ctrl Pts',(-55.8404357399316,9.3173037934771,4.48657761745079));
#34035=CARTESIAN_POINT('Ctrl Pts',(-59.2796040230342,10.,1.49599650170942));
#34036=CARTESIAN_POINT('Ctrl Pts',(-61.,10.,0.));
#34037=CARTESIAN_POINT('Origin',(-61.,0.,-1.11022302462516E-15));
#34038=CARTESIAN_POINT('Origin',(61.,-25.,18.));
#34039=CARTESIAN_POINT('',(56.5,-25.,18.));
#34040=CARTESIAN_POINT('Origin',(-61.,25.,18.));
#34041=CARTESIAN_POINT('',(-65.5,25.,18.));
#34042=CARTESIAN_POINT('Origin',(-61.,-25.,18.));
#34043=CARTESIAN_POINT('',(-65.5,-25.,18.));
#34044=CARTESIAN_POINT('Origin',(61.,25.,18.));
#34045=CARTESIAN_POINT('',(56.5,25.,18.));
#34046=CARTESIAN_POINT('Origin',(-61.,0.,18.));
#34047=CARTESIAN_POINT('',(-71.,1.22464679914735E-15,18.));
#34048=CARTESIAN_POINT('Origin',(61.,0.,18.));
#34049=CARTESIAN_POINT('',(51.,1.22464679914735E-15,18.));
#34050=CARTESIAN_POINT('Origin',(-85.05,0.,0.));
#34051=CARTESIAN_POINT('',(-85.05,-12.05,-1.47569939297256E-15));
#34052=CARTESIAN_POINT('Origin',(108.,10.55,0.));
#34053=CARTESIAN_POINT('Origin',(79.,-27.,-24.));
#34054=CARTESIAN_POINT('',(79.,-14.,-1.71450551880629E-15));
#34055=CARTESIAN_POINT('Origin',(79.,0.,0.));
#34056=CARTESIAN_POINT('Origin',(10.,0.,0.));
#34057=CARTESIAN_POINT('',(10.,-14.,-1.71450551880629E-15));
#34058=CARTESIAN_POINT('Origin',(-43.,-27.,-24.));
#34059=CARTESIAN_POINT('',(-43.,-14.,-1.71450551880629E-15));
#34060=CARTESIAN_POINT('Origin',(-43.,0.,0.));
#34061=CARTESIAN_POINT('Origin',(10.,0.,0.));
#34062=CARTESIAN_POINT('',(10.,-14.,-1.71450551880629E-15));
#34063=CARTESIAN_POINT('Origin',(10.,0.,0.));
#34064=CARTESIAN_POINT('',(10.,-14.,-1.71450551880629E-15));
#56606=UNCERTAINTY_MEASURE_WITH_UNIT(LENGTH_MEASURE(0.01),#56640,
'DISTANCE_ACCURACY_VALUE',
'Maximum model space distance between geometric entities at asserted c
onnectivities');
#56617=UNCERTAINTY_MEASURE_WITH_UNIT(LENGTH_MEASURE(0.01),#56640,
'DISTANCE_ACCURACY_VALUE',
'Maximum model space distance between geometric entities at asserted c
onnectivities');
#56628=(
GEOMETRIC_REPRESENTATION_CONTEXT(3)
GLOBAL_UNCERTAINTY_ASSIGNED_CONTEXT((#56606))
GLOBAL_UNIT_ASSIGNED_CONTEXT((#56640,#56642,#56643))
REPRESENTATION_CONTEXT('','3D')
);
#56639=(
GEOMETRIC_REPRESENTATION_CONTEXT(3)
GLOBAL_UNCERTAINTY_ASSIGNED_CONTEXT((#56617))
GLOBAL_UNIT_ASSIGNED_CONTEXT((#56640,#56642,#56643))
REPRESENTATION_CONTEXT('','3D')
);
#56640=(
LENGTH_UNIT()
NAMED_UNIT(*)
SI_UNIT(.MILLI.,.METRE.)
);
#56642=(
NAMED_UNIT(*)
PLANE_ANGLE_UNIT()
SI_UNIT($,.RADIAN.)
);
#56643=(
NAMED_UNIT(*)
SI_UNIT($,.STERADIAN.)
SOLID_ANGLE_UNIT()
);
#56654=SHAPE_DEFINITION_REPRESENTATION(#56675,#56754);
#56675=PRODUCT_DEFINITION_SHAPE('',$,#56776);
#56754=SHAPE_REPRESENTATION('',(#17818),#56628);
#56765=PRODUCT_DEFINITION_CONTEXT('part definition',#56830,'design');
#56776=PRODUCT_DEFINITION('2026-10-26-00-02-44-429','10_Manifold',#56797,
#56765);
#56797=PRODUCT_DEFINITION_FORMATION('',$,#56842);
#56830=APPLICATION_CONTEXT(
'Core Data for Automotive Mechanical Design Process');
#56831=PRODUCT_CONTEXT('part definition',#56830,'mechanical');
#56842=PRODUCT('2026-10-26-00-02-44-429','10_Manifold',$,(#56831));
#56923=COLOUR_RGB('Off White',0.89,0.88,0.83);
#56924=FILL_AREA_STYLE_COLOUR('',#56923);
#56925=FILL_AREA_STYLE('',(#56924));
#56926=SURFACE_STYLE_FILL_AREA(#56925);
#56927=SURFACE_SIDE_STYLE('',(#56926));
#56928=SURFACE_STYLE_USAGE(.BOTH.,#56927);
#56929=PRESENTATION_STYLE_ASSIGNMENT((#56928));
ENDSEC;
END-ISO-10303-21;
